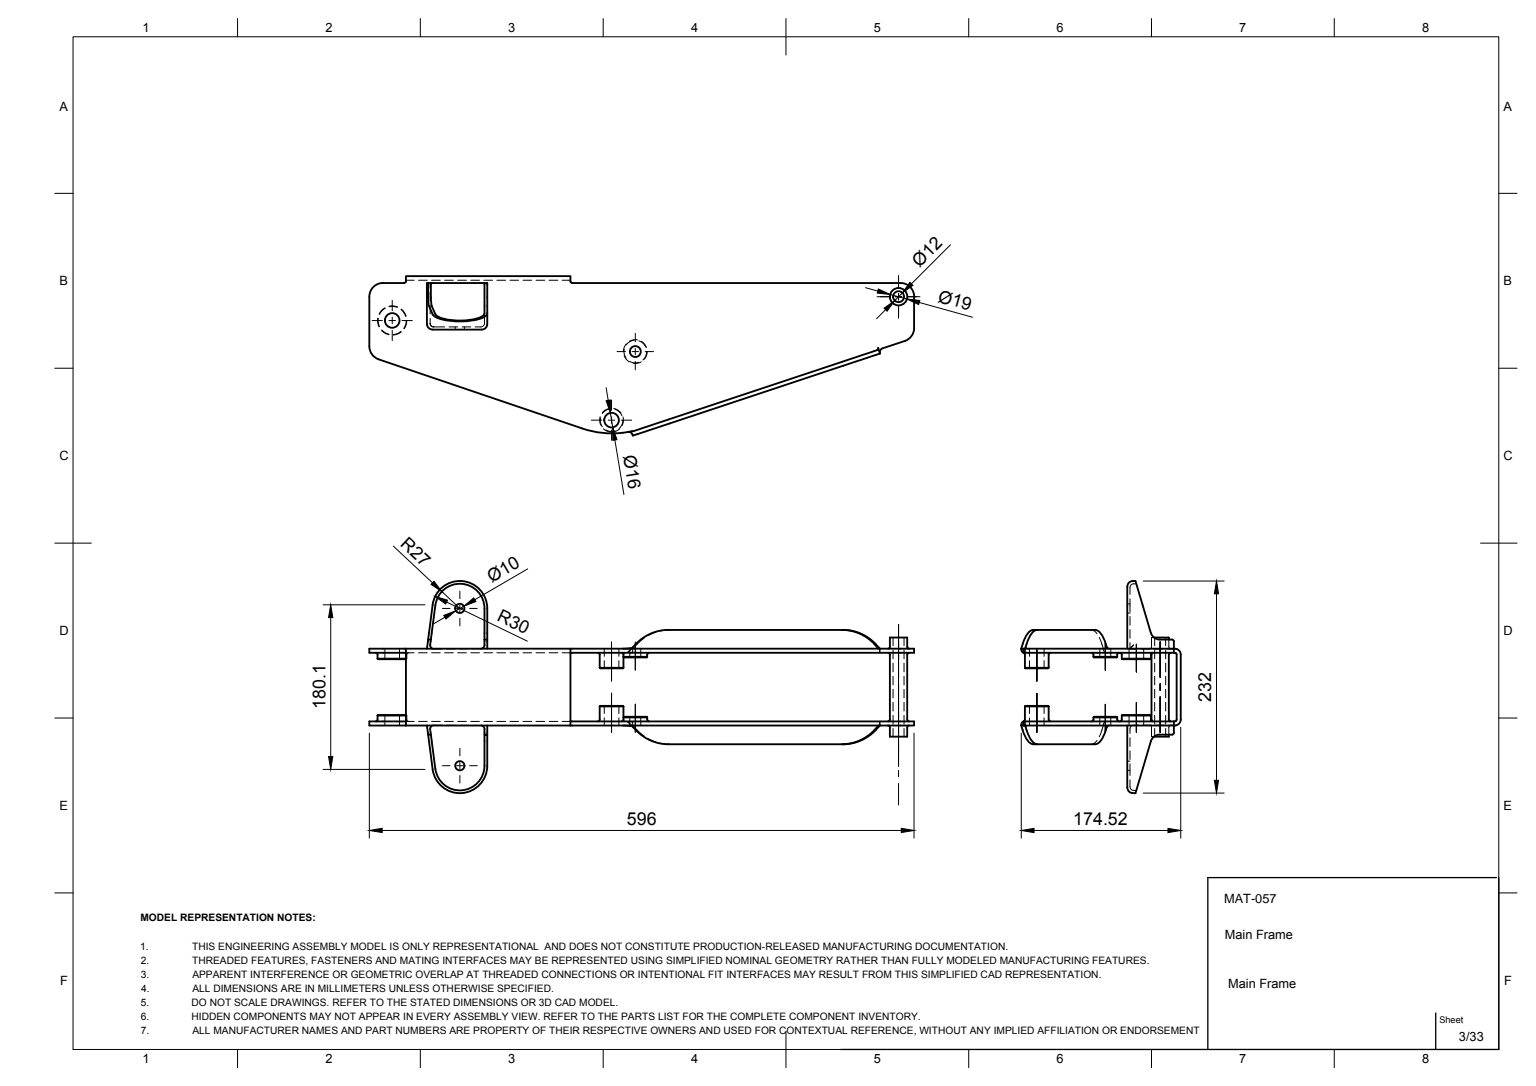
ISO-10303-21;
HEADER;
/* Generated by software containing ST-Developer
 * from STEP Tools, Inc. (www.steptools.com) 
 */

FILE_DESCRIPTION(
/* description */ ('STEP AP214', 'CAx-IF Rec.Pracs.---Representation and Presentation of Product Manufa
cturing Information (PMI)---4.0---2014-10-13'),
/* implementation_level */ '2;1');

FILE_NAME(
/* name */ 'Main Frame.step',
/* time_stamp */ '2026-10-28T23:34:22+01:00',
/* author */ (''),
/* organization */ (''),
/* preprocessor_version */ 'ST-DEVELOPER v20.2',
/* originating_system */ 'Autodesk Translation Framework v15.17.0.0',
/* authorisation */ '');

FILE_SCHEMA (('AP242_MANAGED_MODEL_BASED_3D_ENGINEERING_MIM_LF { 1 0 10303 442 2 1 4 }'));
ENDSEC;

DATA;
#10=MECHANICAL_DESIGN_GEOMETRIC_PRESENTATION_REPRESENTATION('',(#250),#27807);
#206=SHAPE_REPRESENTATION_RELATIONSHIP('SRR','None',#27900,#228);
#228=ADVANCED_BREP_SHAPE_REPRESENTATION('',(#279),#27780);
#250=STYLED_ITEM('',(#28056),#279);
#279=MANIFOLD_SOLID_BREP('Body1',#12026);
#308=(
BOUNDED_SURFACE()
B_SPLINE_SURFACE(3,2,((#18358,#18359,#18360),(#18361,#18362,#18363),(#18364,
#18365,#18366),(#18367,#18368,#18369),(#18370,#18371,#18372),(#18373,#18374,
#18375),(#18376,#18377,#18378),(#18379,#18380,#18381),(#18382,#18383,#18384),
(#18385,#18386,#18387),(#18388,#18389,#18390),(#18391,#18392,#18393)),
 .UNSPECIFIED.,.F.,.F.,.F.)
B_SPLINE_SURFACE_WITH_KNOTS((4,2,2,2,2,4),(3,3),(0.00614272984621533,0.00826669470830694,
0.0093243666888766,0.0103820386694462,0.0124973826305856,0.0146213474926772),
(-5.56138348356354E-6,1.00000862090095),.UNSPECIFIED.)
GEOMETRIC_REPRESENTATION_ITEM()
RATIONAL_B_SPLINE_SURFACE(((1.00000326161464,0.706759768309428,1.00000505596187),
(1.00000294808663,0.734947962870916,1.0000045699493),(1.00000271960407,
0.755490020803058,1.00000421576918),(1.00000249159586,0.775989432119934,
1.00000386232436),(1.00000243486445,0.781089952812372,1.00000377438268),
(1.00000236001445,0.787819451076599,1.00000365835465),(1.00000234158956,
0.789475967918314,1.00000362979347),(1.00000234175209,0.789461355655222,
1.00000363004541),(1.00000241511518,0.782865540172825,1.00000374376852),
(1.00000271619428,0.755796583331183,1.00000421048352),(1.00000294648698,
0.73509178111339,1.00000456746963),(1.00000326163437,0.706757994665561,
1.00000505599245)))
REPRESENTATION_ITEM('')
SURFACE()
);
#309=(
BOUNDED_SURFACE()
B_SPLINE_SURFACE(3,2,((#18394,#18395,#18396),(#18397,#18398,#18399),(#18400,
#18401,#18402),(#18403,#18404,#18405),(#18406,#18407,#18408),(#18409,#18410,
#18411),(#18412,#18413,#18414),(#18415,#18416,#18417),(#18418,#18419,#18420),
(#18421,#18422,#18423),(#18424,#18425,#18426),(#18427,#18428,#18429)),
 .UNSPECIFIED.,.F.,.F.,.F.)
B_SPLINE_SURFACE_WITH_KNOTS((4,2,2,2,2,4),(3,3),(0.0061427298469283,0.00826669470830711,
0.00932436668887678,0.0103820386694465,0.0124973826305858,0.0146213474919646),
(-5.56138389865551E-6,1.00000862090024),.UNSPECIFIED.)
GEOMETRIC_REPRESENTATION_ITEM()
RATIONAL_B_SPLINE_SURFACE(((1.00000326161489,0.706759768337872,1.00000505596145),
(1.00000294808685,0.734947962886857,1.00000456994892),(1.00000271960428,
0.755490020804993,1.00000421576883),(1.00000249159605,0.775989432121355,
1.00000386232404),(1.00000243486463,0.781089952811801,1.00000377438237),
(1.00000236001463,0.787819451077305,1.00000365835434),(1.00000234158974,
0.789475967918561,1.00000362979317),(1.00000234175227,0.789461355654949,
1.00000363004511),(1.00000241511536,0.782865540177451,1.00000374376821),
(1.00000271619448,0.755796583331235,1.00000421048317),(1.0000029464872,
0.735091781130856,1.00000456746925),(1.00000326163462,0.706757994694133,
1.00000505599203)))
REPRESENTATION_ITEM('')
SURFACE()
);
#327=SPHERICAL_SURFACE('',#12617,4.);
#328=SPHERICAL_SURFACE('',#12619,4.);
#335=FACE_BOUND('',#2001,.T.);
#336=FACE_BOUND('',#2002,.T.);
#337=FACE_BOUND('',#2003,.T.);
#338=FACE_BOUND('',#2004,.T.);
#339=FACE_BOUND('',#2005,.T.);
#340=FACE_BOUND('',#2007,.T.);
#341=FACE_BOUND('',#2008,.T.);
#342=FACE_BOUND('',#2009,.T.);
#343=FACE_BOUND('',#2014,.T.);
#344=FACE_BOUND('',#2015,.T.);
#345=FACE_BOUND('',#2016,.T.);
#346=FACE_BOUND('',#2017,.T.);
#347=FACE_BOUND('',#2018,.T.);
#348=FACE_BOUND('',#2024,.T.);
#349=FACE_BOUND('',#2029,.T.);
#350=FACE_BOUND('',#2034,.T.);
#351=FACE_BOUND('',#2051,.T.);
#352=FACE_BOUND('',#2053,.T.);
#353=FACE_BOUND('',#2055,.T.);
#354=FACE_BOUND('',#2061,.T.);
#355=FACE_BOUND('',#2062,.T.);
#356=FACE_BOUND('',#2063,.T.);
#357=FACE_BOUND('',#2065,.T.);
#358=FACE_BOUND('',#2067,.T.);
#359=FACE_BOUND('',#2072,.T.);
#360=FACE_BOUND('',#2083,.T.);
#361=FACE_BOUND('',#2085,.T.);
#362=FACE_BOUND('',#2087,.T.);
#448=PLANE('',#12425);
#449=PLANE('',#12427);
#450=PLANE('',#12428);
#451=PLANE('',#12429);
#452=PLANE('',#12431);
#453=PLANE('',#12432);
#454=PLANE('',#12440);
#455=PLANE('',#12443);
#456=PLANE('',#12444);
#457=PLANE('',#12451);
#458=PLANE('',#12452);
#459=PLANE('',#12453);
#460=PLANE('',#12455);
#461=PLANE('',#12457);
#462=PLANE('',#12466);
#463=PLANE('',#12477);
#464=PLANE('',#12478);
#465=PLANE('',#12482);
#466=PLANE('',#12493);
#467=PLANE('',#12494);
#468=PLANE('',#12495);
#469=PLANE('',#12496);
#470=PLANE('',#12497);
#471=PLANE('',#12498);
#472=PLANE('',#12503);
#473=PLANE('',#12506);
#474=PLANE('',#12508);
#475=PLANE('',#12511);
#476=PLANE('',#12513);
#477=PLANE('',#12515);
#478=PLANE('',#12519);
#479=PLANE('',#12521);
#480=PLANE('',#12529);
#481=PLANE('',#12530);
#482=PLANE('',#12533);
#483=PLANE('',#12535);
#484=PLANE('',#12537);
#485=PLANE('',#12540);
#486=PLANE('',#12543);
#487=PLANE('',#12544);
#488=PLANE('',#12545);
#489=PLANE('',#12546);
#490=PLANE('',#12547);
#491=PLANE('',#12548);
#492=PLANE('',#12549);
#493=PLANE('',#12550);
#494=PLANE('',#12558);
#495=PLANE('',#12559);
#496=PLANE('',#12560);
#497=PLANE('',#12562);
#498=PLANE('',#12564);
#499=PLANE('',#12566);
#500=PLANE('',#12571);
#501=PLANE('',#12573);
#502=PLANE('',#12576);
#503=PLANE('',#12577);
#504=PLANE('',#12579);
#505=PLANE('',#12582);
#506=PLANE('',#12583);
#507=PLANE('',#12584);
#508=PLANE('',#12585);
#509=PLANE('',#12588);
#510=PLANE('',#12589);
#511=PLANE('',#12591);
#512=PLANE('',#12592);
#513=PLANE('',#12597);
#747=ELLIPSE('',#12376,5.6568542494854,3.99999999999488);
#748=ELLIPSE('',#12390,28.164698545175,26.9999999999996);
#749=ELLIPSE('',#12421,31.2941094946442,30.0000000000042);
#750=ELLIPSE('',#12435,141.421352252718,99.9999944851797);
#751=ELLIPSE('',#12449,10.0848897519878,9.99999999999638);
#752=ELLIPSE('',#12450,10.0848897519895,9.99999999999823);
#753=ELLIPSE('',#12456,2.01697795039841,2.0000000000002);
#754=ELLIPSE('',#12465,6.05093385119014,5.9999999999955);
#755=ELLIPSE('',#12492,6.05093385118888,5.99999999999402);
#756=ELLIPSE('',#12502,31.2941094946394,29.9999999999999);
#757=ELLIPSE('',#12504,10.0848897519875,9.99999999999656);
#758=ELLIPSE('',#12505,2.01697795039468,1.99999999999602);
#759=ELLIPSE('',#12510,10.084889751988,9.99999999999652);
#760=ELLIPSE('',#12512,28.1646985451758,27.);
#761=ELLIPSE('',#12520,2.01697795039476,1.99999999999607);
#762=ELLIPSE('',#12523,141.421350791142,99.9999924642367);
#763=ELLIPSE('',#12534,2.82842712474556,1.9999999999995);
#764=ELLIPSE('',#12538,2.8284271247638,2.00000000001808);
#765=ELLIPSE('',#12539,6.36396103068019,4.50000000000073);
#766=ELLIPSE('',#12561,4.00607672981957,4.00312101599644);
#767=ELLIPSE('',#12565,2.01697795039961,2.00000000000168);
#768=ELLIPSE('',#12574,6.36396103067894,4.49999999999996);
#769=ELLIPSE('',#12575,2.82842712478915,2.00000000005605);
#770=ELLIPSE('',#12578,2.82842712474301,1.99999999999741);
#771=ELLIPSE('',#12607,5.65685424949513,4.00000000000238);
#811=TOROIDAL_SURFACE('',#12321,24.,6.);
#812=TOROIDAL_SURFACE('',#12326,18.,2.);
#813=TOROIDAL_SURFACE('',#12330,15.,2.);
#814=TOROIDAL_SURFACE('',#12334,15.,2.);
#815=TOROIDAL_SURFACE('',#12338,18.,2.);
#816=TOROIDAL_SURFACE('',#12342,15.,2.);
#817=TOROIDAL_SURFACE('',#12348,15.,2.);
#818=TOROIDAL_SURFACE('',#12354,11.5,2.);
#819=TOROIDAL_SURFACE('',#12359,11.5,2.);
#820=TOROIDAL_SURFACE('',#12363,11.5,2.);
#821=TOROIDAL_SURFACE('',#12368,11.5,2.);
#822=TOROIDAL_SURFACE('',#12378,23.,4.);
#823=TOROIDAL_SURFACE('',#12625,23.,4.);
#824=TOROIDAL_SURFACE('',#12640,24.,6.);
#850=B_SPLINE_CURVE_WITH_KNOTS('',3,(#17467,#17468,#17469,#17470,#17471,
#17472,#17473,#17474,#17475,#17476,#17477,#17478),.UNSPECIFIED.,.F.,.F.,
(4,2,2,2,2,4),(2.0099992972745,2.20224824152656,2.28793503314165,2.37362182475674,
2.53832634192652,2.7030308590963),.UNSPECIFIED.);
#851=B_SPLINE_CURVE_WITH_KNOTS('',3,(#17597,#17598,#17599,#17600,#17601,
#17602,#17603,#17604,#17605,#17606,#17607,#17608),.UNSPECIFIED.,.F.,.F.,
(4,2,2,2,2,4),(0.,0.00181440406025865,0.00272160609038796,0.00362880812051727,
0.00544321218077591,0.00725761624103455),.UNSPECIFIED.);
#852=B_SPLINE_CURVE_WITH_KNOTS('',3,(#17643,#17644,#17645,#17646,#17647,
#17648,#17649,#17650,#17651,#17652,#17653,#17654),.UNSPECIFIED.,.F.,.F.,
(4,2,2,2,2,4),(0.,0.00181440406025865,0.00272160609038798,0.0036288081205173,
0.00544321218077593,0.00725761624103456),.UNSPECIFIED.);
#853=B_SPLINE_CURVE_WITH_KNOTS('',3,(#17772,#17773,#17774,#17775,#17776,
#17777),.UNSPECIFIED.,.F.,.F.,(4,2,4),(-1.89448158063908,-0.947240790319523,
-0.943407967638861),.UNSPECIFIED.);
#854=B_SPLINE_CURVE_WITH_KNOTS('',3,(#18063,#18064,#18065,#18066,#18067,
#18068),.UNSPECIFIED.,.F.,.F.,(4,2,4),(-4.54637383394205,-4.54254101126139,
-3.59530022094183),.UNSPECIFIED.);
#855=B_SPLINE_CURVE_WITH_KNOTS('',3,(#18285,#18286,#18287,#18288,#18289,
#18290,#18291,#18292,#18293,#18294),.UNSPECIFIED.,.F.,.F.,(4,2,2,2,4),(-1.65528023567133,
-1.60355895330957,-1.50636781568743,-1.40917667806529,-1.31726787147769),
 .UNSPECIFIED.);
#856=B_SPLINE_CURVE_WITH_KNOTS('',3,(#18296,#18297,#18298,#18299,#18300,
#18301,#18302,#18303,#18304,#18305),.UNSPECIFIED.,.F.,.F.,(4,2,2,2,4),(-0.723638776454986,
-0.631729969867392,-0.53453883224525,-0.437347694623109,-0.385626412261347),
 .UNSPECIFIED.);
#857=B_SPLINE_CURVE_WITH_KNOTS('',3,(#18306,#18307,#18308,#18309,#18310,
#18311,#18312,#18313,#18314,#18315,#18316,#18317),.UNSPECIFIED.,.F.,.F.,
(4,2,2,2,2,4),(0.207978724543637,0.400227668795699,0.48591446041079,0.57160125202588,
0.736305769195657,0.901010286365433),.UNSPECIFIED.);
#858=B_SPLINE_CURVE_WITH_KNOTS('',3,(#18319,#18320,#18321,#18322,#18323,
#18324,#18325,#18326),.UNSPECIFIED.,.F.,.F.,(4,2,2,4),(0.724350563126704,
0.774624716441459,0.824898869756215,0.828883959825179),.UNSPECIFIED.);
#859=B_SPLINE_CURVE_WITH_KNOTS('',3,(#18327,#18328,#18329,#18330,#18331,
#18332,#18333,#18334),.UNSPECIFIED.,.F.,.F.,(4,2,2,4),(1.23194128218264,
1.2359263722516,1.28620052556636,1.33647467888111),.UNSPECIFIED.);
#860=B_SPLINE_CURVE_WITH_KNOTS('',3,(#18336,#18337,#18338,#18339,#18340,
#18341,#18342,#18343),.UNSPECIFIED.,.F.,.F.,(4,2,2,4),(-0.306062057877202,
-0.255787904562446,-0.205513751247691,-0.201528661178732),.UNSPECIFIED.);
#861=B_SPLINE_CURVE_WITH_KNOTS('',3,(#18344,#18345,#18346,#18347,#18348,
#18349,#18350,#18351),.UNSPECIFIED.,.F.,.F.,(4,2,2,4),(0.201528661178729,
0.205513751247691,0.255787904562446,0.306062057877201),.UNSPECIFIED.);
#862=B_SPLINE_CURVE_WITH_KNOTS('',3,(#18438,#18439,#18440,#18441,#18442,
#18443),.UNSPECIFIED.,.F.,.F.,(4,2,4),(-0.302135903177322,-0.22673410522417,
-0.201580663771353),.UNSPECIFIED.);
#863=B_SPLINE_CURVE_WITH_KNOTS('',3,(#18445,#18446,#18447,#18448,#18449,
#18450),.UNSPECIFIED.,.F.,.F.,(4,2,4),(-0.409607477693974,-0.384454036241157,
-0.309052238288002),.UNSPECIFIED.);
#864=B_SPLINE_CURVE_WITH_KNOTS('',3,(#18452,#18453,#18454,#18455,#18456,
#18457),.UNSPECIFIED.,.F.,.F.,(4,2,4),(-0.302135903177326,-0.226734105224171,
-0.201580663771353),.UNSPECIFIED.);
#865=B_SPLINE_CURVE_WITH_KNOTS('',3,(#18459,#18460,#18461,#18462,#18463,
#18464),.UNSPECIFIED.,.F.,.F.,(4,2,4),(-0.409607477693974,-0.384454036241154,
-0.309052238288002),.UNSPECIFIED.);
#975=CYLINDRICAL_SURFACE('',#12318,4.5);
#976=CYLINDRICAL_SURFACE('',#12373,4.);
#977=CYLINDRICAL_SURFACE('',#12383,6.00000000000001);
#978=CYLINDRICAL_SURFACE('',#12386,13.);
#979=CYLINDRICAL_SURFACE('',#12387,13.);
#980=CYLINDRICAL_SURFACE('',#12388,16.);
#981=CYLINDRICAL_SURFACE('',#12389,27.);
#982=CYLINDRICAL_SURFACE('',#12391,9.50000000000001);
#983=CYLINDRICAL_SURFACE('',#12393,5.99999999999999);
#984=CYLINDRICAL_SURFACE('',#12396,8.00000000000001);
#985=CYLINDRICAL_SURFACE('',#12399,7.99999999999999);
#986=CYLINDRICAL_SURFACE('',#12402,13.);
#987=CYLINDRICAL_SURFACE('',#12403,13.);
#988=CYLINDRICAL_SURFACE('',#12404,16.);
#989=CYLINDRICAL_SURFACE('',#12405,9.50000000000001);
#990=CYLINDRICAL_SURFACE('',#12407,5.99999999999999);
#991=CYLINDRICAL_SURFACE('',#12410,8.00000000000001);
#992=CYLINDRICAL_SURFACE('',#12413,7.99999999999999);
#993=CYLINDRICAL_SURFACE('',#12416,9.50000000000001);
#994=CYLINDRICAL_SURFACE('',#12417,5.);
#995=CYLINDRICAL_SURFACE('',#12420,30.);
#996=CYLINDRICAL_SURFACE('',#12422,5.);
#997=CYLINDRICAL_SURFACE('',#12434,100.);
#998=CYLINDRICAL_SURFACE('',#12445,10.);
#999=CYLINDRICAL_SURFACE('',#12448,10.);
#1000=CYLINDRICAL_SURFACE('',#12479,10.);
#1001=CYLINDRICAL_SURFACE('',#12500,30.);
#1002=CYLINDRICAL_SURFACE('',#12509,10.);
#1003=CYLINDRICAL_SURFACE('',#12517,27.);
#1004=CYLINDRICAL_SURFACE('',#12522,100.);
#1005=CYLINDRICAL_SURFACE('',#12525,15.);
#1006=CYLINDRICAL_SURFACE('',#12526,15.);
#1007=CYLINDRICAL_SURFACE('',#12527,15.);
#1008=CYLINDRICAL_SURFACE('',#12528,15.);
#1009=CYLINDRICAL_SURFACE('',#12567,15.);
#1010=CYLINDRICAL_SURFACE('',#12568,15.);
#1011=CYLINDRICAL_SURFACE('',#12569,15.);
#1012=CYLINDRICAL_SURFACE('',#12570,15.);
#1013=CYLINDRICAL_SURFACE('',#12602,53.);
#1014=CYLINDRICAL_SURFACE('',#12603,53.);
#1015=CYLINDRICAL_SURFACE('',#12604,53.);
#1016=CYLINDRICAL_SURFACE('',#12605,53.);
#1017=CYLINDRICAL_SURFACE('',#12606,4.);
#1018=CYLINDRICAL_SURFACE('',#12608,4.);
#1019=CYLINDRICAL_SURFACE('',#12609,4.00000000000001);
#1020=CYLINDRICAL_SURFACE('',#12610,4.);
#1021=CYLINDRICAL_SURFACE('',#12612,4.);
#1022=CYLINDRICAL_SURFACE('',#12614,3.99999999999998);
#1023=CYLINDRICAL_SURFACE('',#12621,4.);
#1024=CYLINDRICAL_SURFACE('',#12623,4.);
#1025=CYLINDRICAL_SURFACE('',#12626,4.);
#1026=CYLINDRICAL_SURFACE('',#12627,4.);
#1027=CYLINDRICAL_SURFACE('',#12628,2.);
#1028=CYLINDRICAL_SURFACE('',#12629,2.);
#1029=CYLINDRICAL_SURFACE('',#12630,2.);
#1030=CYLINDRICAL_SURFACE('',#12631,2.);
#1031=CYLINDRICAL_SURFACE('',#12632,1.99999999999999);
#1032=CYLINDRICAL_SURFACE('',#12633,1.99999999999999);
#1033=CYLINDRICAL_SURFACE('',#12634,2.);
#1034=CYLINDRICAL_SURFACE('',#12635,2.);
#1035=CYLINDRICAL_SURFACE('',#12636,6.00000000000001);
#1036=CYLINDRICAL_SURFACE('',#12637,5.99999999999999);
#1037=CYLINDRICAL_SURFACE('',#12638,6.00000000000001);
#1038=CYLINDRICAL_SURFACE('',#12642,5.99999999999999);
#1039=CYLINDRICAL_SURFACE('',#12643,2.);
#1040=CYLINDRICAL_SURFACE('',#12644,2.);
#1041=CYLINDRICAL_SURFACE('',#12645,2.);
#1042=CYLINDRICAL_SURFACE('',#12646,2.);
#1043=CYLINDRICAL_SURFACE('',#12647,4.5);
#1044=CYLINDRICAL_SURFACE('',#12648,4.5);
#1045=CYLINDRICAL_SURFACE('',#12649,4.5);
#1046=CYLINDRICAL_SURFACE('',#12650,6.50000000000001);
#1047=CYLINDRICAL_SURFACE('',#12651,6.50000000000001);
#1247=FACE_OUTER_BOUND('',#1944,.T.);
#1248=FACE_OUTER_BOUND('',#1945,.T.);
#1249=FACE_OUTER_BOUND('',#1946,.T.);
#1250=FACE_OUTER_BOUND('',#1947,.T.);
#1251=FACE_OUTER_BOUND('',#1948,.T.);
#1252=FACE_OUTER_BOUND('',#1949,.T.);
#1253=FACE_OUTER_BOUND('',#1950,.T.);
#1254=FACE_OUTER_BOUND('',#1951,.T.);
#1255=FACE_OUTER_BOUND('',#1952,.T.);
#1256=FACE_OUTER_BOUND('',#1953,.T.);
#1257=FACE_OUTER_BOUND('',#1954,.T.);
#1258=FACE_OUTER_BOUND('',#1955,.T.);
#1259=FACE_OUTER_BOUND('',#1956,.T.);
#1260=FACE_OUTER_BOUND('',#1957,.T.);
#1261=FACE_OUTER_BOUND('',#1958,.T.);
#1262=FACE_OUTER_BOUND('',#1959,.T.);
#1263=FACE_OUTER_BOUND('',#1960,.T.);
#1264=FACE_OUTER_BOUND('',#1961,.T.);
#1265=FACE_OUTER_BOUND('',#1962,.T.);
#1266=FACE_OUTER_BOUND('',#1963,.T.);
#1267=FACE_OUTER_BOUND('',#1964,.T.);
#1268=FACE_OUTER_BOUND('',#1965,.T.);
#1269=FACE_OUTER_BOUND('',#1966,.T.);
#1270=FACE_OUTER_BOUND('',#1967,.T.);
#1271=FACE_OUTER_BOUND('',#1968,.T.);
#1272=FACE_OUTER_BOUND('',#1969,.T.);
#1273=FACE_OUTER_BOUND('',#1970,.T.);
#1274=FACE_OUTER_BOUND('',#1971,.T.);
#1275=FACE_OUTER_BOUND('',#1972,.T.);
#1276=FACE_OUTER_BOUND('',#1973,.T.);
#1277=FACE_OUTER_BOUND('',#1974,.T.);
#1278=FACE_OUTER_BOUND('',#1975,.T.);
#1279=FACE_OUTER_BOUND('',#1976,.T.);
#1280=FACE_OUTER_BOUND('',#1977,.T.);
#1281=FACE_OUTER_BOUND('',#1978,.T.);
#1282=FACE_OUTER_BOUND('',#1979,.T.);
#1283=FACE_OUTER_BOUND('',#1980,.T.);
#1284=FACE_OUTER_BOUND('',#1981,.T.);
#1285=FACE_OUTER_BOUND('',#1982,.T.);
#1286=FACE_OUTER_BOUND('',#1983,.T.);
#1287=FACE_OUTER_BOUND('',#1984,.T.);
#1288=FACE_OUTER_BOUND('',#1985,.T.);
#1289=FACE_OUTER_BOUND('',#1986,.T.);
#1290=FACE_OUTER_BOUND('',#1987,.T.);
#1291=FACE_OUTER_BOUND('',#1988,.T.);
#1292=FACE_OUTER_BOUND('',#1989,.T.);
#1293=FACE_OUTER_BOUND('',#1990,.T.);
#1294=FACE_OUTER_BOUND('',#1991,.T.);
#1295=FACE_OUTER_BOUND('',#1992,.T.);
#1296=FACE_OUTER_BOUND('',#1993,.T.);
#1297=FACE_OUTER_BOUND('',#1994,.T.);
#1298=FACE_OUTER_BOUND('',#1995,.T.);
#1299=FACE_OUTER_BOUND('',#1996,.T.);
#1300=FACE_OUTER_BOUND('',#1997,.T.);
#1301=FACE_OUTER_BOUND('',#1998,.T.);
#1302=FACE_OUTER_BOUND('',#1999,.T.);
#1303=FACE_OUTER_BOUND('',#2000,.T.);
#1304=FACE_OUTER_BOUND('',#2006,.T.);
#1305=FACE_OUTER_BOUND('',#2010,.T.);
#1306=FACE_OUTER_BOUND('',#2011,.T.);
#1307=FACE_OUTER_BOUND('',#2012,.T.);
#1308=FACE_OUTER_BOUND('',#2013,.T.);
#1309=FACE_OUTER_BOUND('',#2019,.T.);
#1310=FACE_OUTER_BOUND('',#2020,.T.);
#1311=FACE_OUTER_BOUND('',#2021,.T.);
#1312=FACE_OUTER_BOUND('',#2022,.T.);
#1313=FACE_OUTER_BOUND('',#2023,.T.);
#1314=FACE_OUTER_BOUND('',#2025,.T.);
#1315=FACE_OUTER_BOUND('',#2026,.T.);
#1316=FACE_OUTER_BOUND('',#2027,.T.);
#1317=FACE_OUTER_BOUND('',#2028,.T.);
#1318=FACE_OUTER_BOUND('',#2030,.T.);
#1319=FACE_OUTER_BOUND('',#2031,.T.);
#1320=FACE_OUTER_BOUND('',#2032,.T.);
#1321=FACE_OUTER_BOUND('',#2033,.T.);
#1322=FACE_OUTER_BOUND('',#2035,.T.);
#1323=FACE_OUTER_BOUND('',#2036,.T.);
#1324=FACE_OUTER_BOUND('',#2037,.T.);
#1325=FACE_OUTER_BOUND('',#2038,.T.);
#1326=FACE_OUTER_BOUND('',#2039,.T.);
#1327=FACE_OUTER_BOUND('',#2040,.T.);
#1328=FACE_OUTER_BOUND('',#2041,.T.);
#1329=FACE_OUTER_BOUND('',#2042,.T.);
#1330=FACE_OUTER_BOUND('',#2043,.T.);
#1331=FACE_OUTER_BOUND('',#2044,.T.);
#1332=FACE_OUTER_BOUND('',#2045,.T.);
#1333=FACE_OUTER_BOUND('',#2046,.T.);
#1334=FACE_OUTER_BOUND('',#2047,.T.);
#1335=FACE_OUTER_BOUND('',#2048,.T.);
#1336=FACE_OUTER_BOUND('',#2049,.T.);
#1337=FACE_OUTER_BOUND('',#2050,.T.);
#1338=FACE_OUTER_BOUND('',#2052,.T.);
#1339=FACE_OUTER_BOUND('',#2054,.T.);
#1340=FACE_OUTER_BOUND('',#2056,.T.);
#1341=FACE_OUTER_BOUND('',#2057,.T.);
#1342=FACE_OUTER_BOUND('',#2058,.T.);
#1343=FACE_OUTER_BOUND('',#2059,.T.);
#1344=FACE_OUTER_BOUND('',#2060,.T.);
#1345=FACE_OUTER_BOUND('',#2064,.T.);
#1346=FACE_OUTER_BOUND('',#2066,.T.);
#1347=FACE_OUTER_BOUND('',#2068,.T.);
#1348=FACE_OUTER_BOUND('',#2069,.T.);
#1349=FACE_OUTER_BOUND('',#2070,.T.);
#1350=FACE_OUTER_BOUND('',#2071,.T.);
#1351=FACE_OUTER_BOUND('',#2073,.T.);
#1352=FACE_OUTER_BOUND('',#2074,.T.);
#1353=FACE_OUTER_BOUND('',#2075,.T.);
#1354=FACE_OUTER_BOUND('',#2076,.T.);
#1355=FACE_OUTER_BOUND('',#2077,.T.);
#1356=FACE_OUTER_BOUND('',#2078,.T.);
#1357=FACE_OUTER_BOUND('',#2079,.T.);
#1358=FACE_OUTER_BOUND('',#2080,.T.);
#1359=FACE_OUTER_BOUND('',#2081,.T.);
#1360=FACE_OUTER_BOUND('',#2082,.T.);
#1361=FACE_OUTER_BOUND('',#2084,.T.);
#1362=FACE_OUTER_BOUND('',#2086,.T.);
#1363=FACE_OUTER_BOUND('',#2088,.T.);
#1364=FACE_OUTER_BOUND('',#2089,.T.);
#1365=FACE_OUTER_BOUND('',#2090,.T.);
#1366=FACE_OUTER_BOUND('',#2091,.T.);
#1367=FACE_OUTER_BOUND('',#2092,.T.);
#1368=FACE_OUTER_BOUND('',#2093,.T.);
#1369=FACE_OUTER_BOUND('',#2094,.T.);
#1370=FACE_OUTER_BOUND('',#2095,.T.);
#1371=FACE_OUTER_BOUND('',#2096,.T.);
#1372=FACE_OUTER_BOUND('',#2097,.T.);
#1373=FACE_OUTER_BOUND('',#2098,.T.);
#1374=FACE_OUTER_BOUND('',#2099,.T.);
#1375=FACE_OUTER_BOUND('',#2100,.T.);
#1376=FACE_OUTER_BOUND('',#2101,.T.);
#1377=FACE_OUTER_BOUND('',#2102,.T.);
#1378=FACE_OUTER_BOUND('',#2103,.T.);
#1379=FACE_OUTER_BOUND('',#2104,.T.);
#1380=FACE_OUTER_BOUND('',#2105,.T.);
#1381=FACE_OUTER_BOUND('',#2106,.T.);
#1382=FACE_OUTER_BOUND('',#2107,.T.);
#1383=FACE_OUTER_BOUND('',#2108,.T.);
#1384=FACE_OUTER_BOUND('',#2109,.T.);
#1385=FACE_OUTER_BOUND('',#2110,.T.);
#1386=FACE_OUTER_BOUND('',#2111,.T.);
#1387=FACE_OUTER_BOUND('',#2112,.T.);
#1388=FACE_OUTER_BOUND('',#2113,.T.);
#1389=FACE_OUTER_BOUND('',#2114,.T.);
#1390=FACE_OUTER_BOUND('',#2115,.T.);
#1391=FACE_OUTER_BOUND('',#2116,.T.);
#1392=FACE_OUTER_BOUND('',#2117,.T.);
#1393=FACE_OUTER_BOUND('',#2118,.T.);
#1394=FACE_OUTER_BOUND('',#2119,.T.);
#1395=FACE_OUTER_BOUND('',#2120,.T.);
#1396=FACE_OUTER_BOUND('',#2121,.T.);
#1397=FACE_OUTER_BOUND('',#2122,.T.);
#1398=FACE_OUTER_BOUND('',#2123,.T.);
#1399=FACE_OUTER_BOUND('',#2124,.T.);
#1400=FACE_OUTER_BOUND('',#2125,.T.);
#1401=FACE_OUTER_BOUND('',#2126,.T.);
#1402=FACE_OUTER_BOUND('',#2127,.T.);
#1403=FACE_OUTER_BOUND('',#2128,.T.);
#1404=FACE_OUTER_BOUND('',#2129,.T.);
#1405=FACE_OUTER_BOUND('',#2130,.T.);
#1406=FACE_OUTER_BOUND('',#2131,.T.);
#1407=FACE_OUTER_BOUND('',#2132,.T.);
#1408=FACE_OUTER_BOUND('',#2133,.T.);
#1409=FACE_OUTER_BOUND('',#2134,.T.);
#1944=EDGE_LOOP('',(#7851,#7852,#7853,#7854));
#1945=EDGE_LOOP('',(#7855,#7856,#7857,#7858));
#1946=EDGE_LOOP('',(#7859,#7860,#7861,#7862));
#1947=EDGE_LOOP('',(#7863,#7864,#7865,#7866));
#1948=EDGE_LOOP('',(#7867,#7868,#7869,#7870));
#1949=EDGE_LOOP('',(#7871,#7872,#7873,#7874));
#1950=EDGE_LOOP('',(#7875,#7876,#7877,#7878,#7879));
#1951=EDGE_LOOP('',(#7880,#7881,#7882,#7883));
#1952=EDGE_LOOP('',(#7884,#7885,#7886,#7887));
#1953=EDGE_LOOP('',(#7888,#7889,#7890,#7891));
#1954=EDGE_LOOP('',(#7892,#7893,#7894,#7895));
#1955=EDGE_LOOP('',(#7896,#7897,#7898,#7899));
#1956=EDGE_LOOP('',(#7900,#7901,#7902,#7903,#7904));
#1957=EDGE_LOOP('',(#7905,#7906,#7907,#7908,#7909));
#1958=EDGE_LOOP('',(#7910,#7911,#7912,#7913,#7914));
#1959=EDGE_LOOP('',(#7915,#7916,#7917,#7918));
#1960=EDGE_LOOP('',(#7919,#7920,#7921,#7922,#7923));
#1961=EDGE_LOOP('',(#7924,#7925,#7926,#7927,#7928));
#1962=EDGE_LOOP('',(#7929,#7930,#7931,#7932,#7933,#7934));
#1963=EDGE_LOOP('',(#7935,#7936,#7937,#7938));
#1964=EDGE_LOOP('',(#7939,#7940,#7941,#7942));
#1965=EDGE_LOOP('',(#7943,#7944,#7945,#7946));
#1966=EDGE_LOOP('',(#7947,#7948,#7949,#7950,#7951,#7952));
#1967=EDGE_LOOP('',(#7953,#7954,#7955,#7956));
#1968=EDGE_LOOP('',(#7957,#7958,#7959,#7960));
#1969=EDGE_LOOP('',(#7961,#7962,#7963,#7964,#7965));
#1970=EDGE_LOOP('',(#7966,#7967,#7968,#7969));
#1971=EDGE_LOOP('',(#7970,#7971,#7972,#7973));
#1972=EDGE_LOOP('',(#7974,#7975,#7976,#7977));
#1973=EDGE_LOOP('',(#7978,#7979,#7980,#7981));
#1974=EDGE_LOOP('',(#7982,#7983,#7984,#7985,#7986,#7987));
#1975=EDGE_LOOP('',(#7988,#7989,#7990,#7991));
#1976=EDGE_LOOP('',(#7992,#7993,#7994,#7995,#7996));
#1977=EDGE_LOOP('',(#7997,#7998,#7999,#8000));
#1978=EDGE_LOOP('',(#8001,#8002,#8003,#8004));
#1979=EDGE_LOOP('',(#8005,#8006,#8007,#8008));
#1980=EDGE_LOOP('',(#8009,#8010,#8011,#8012,#8013));
#1981=EDGE_LOOP('',(#8014,#8015,#8016,#8017));
#1982=EDGE_LOOP('',(#8018,#8019,#8020,#8021));
#1983=EDGE_LOOP('',(#8022,#8023,#8024,#8025));
#1984=EDGE_LOOP('',(#8026,#8027,#8028,#8029,#8030));
#1985=EDGE_LOOP('',(#8031,#8032,#8033,#8034));
#1986=EDGE_LOOP('',(#8035,#8036,#8037,#8038,#8039));
#1987=EDGE_LOOP('',(#8040,#8041,#8042,#8043,#8044));
#1988=EDGE_LOOP('',(#8045,#8046,#8047,#8048));
#1989=EDGE_LOOP('',(#8049,#8050,#8051,#8052,#8053));
#1990=EDGE_LOOP('',(#8054,#8055,#8056,#8057,#8058,#8059,#8060,#8061));
#1991=EDGE_LOOP('',(#8062,#8063,#8064,#8065,#8066,#8067));
#1992=EDGE_LOOP('',(#8068,#8069,#8070,#8071));
#1993=EDGE_LOOP('',(#8072,#8073,#8074,#8075,#8076,#8077,#8078,#8079));
#1994=EDGE_LOOP('',(#8080,#8081,#8082,#8083));
#1995=EDGE_LOOP('',(#8084,#8085,#8086,#8087));
#1996=EDGE_LOOP('',(#8088,#8089,#8090,#8091));
#1997=EDGE_LOOP('',(#8092,#8093,#8094,#8095));
#1998=EDGE_LOOP('',(#8096,#8097,#8098,#8099,#8100,#8101,#8102,#8103));
#1999=EDGE_LOOP('',(#8104,#8105,#8106,#8107,#8108,#8109,#8110,#8111));
#2000=EDGE_LOOP('',(#8112,#8113,#8114,#8115,#8116,#8117,#8118,#8119,#8120,
#8121,#8122,#8123,#8124,#8125,#8126,#8127,#8128));
#2001=EDGE_LOOP('',(#8129));
#2002=EDGE_LOOP('',(#8130));
#2003=EDGE_LOOP('',(#8131));
#2004=EDGE_LOOP('',(#8132));
#2005=EDGE_LOOP('',(#8133,#8134,#8135,#8136,#8137,#8138,#8139,#8140));
#2006=EDGE_LOOP('',(#8141,#8142,#8143,#8144,#8145,#8146,#8147,#8148,#8149,
#8150,#8151,#8152,#8153,#8154,#8155,#8156,#8157,#8158,#8159));
#2007=EDGE_LOOP('',(#8160));
#2008=EDGE_LOOP('',(#8161));
#2009=EDGE_LOOP('',(#8162));
#2010=EDGE_LOOP('',(#8163,#8164,#8165,#8166));
#2011=EDGE_LOOP('',(#8167,#8168,#8169,#8170));
#2012=EDGE_LOOP('',(#8171,#8172,#8173,#8174));
#2013=EDGE_LOOP('',(#8175,#8176,#8177,#8178,#8179,#8180,#8181,#8182,#8183,
#8184,#8185,#8186,#8187,#8188,#8189,#8190,#8191));
#2014=EDGE_LOOP('',(#8192));
#2015=EDGE_LOOP('',(#8193));
#2016=EDGE_LOOP('',(#8194));
#2017=EDGE_LOOP('',(#8195));
#2018=EDGE_LOOP('',(#8196,#8197,#8198,#8199,#8200,#8201,#8202,#8203));
#2019=EDGE_LOOP('',(#8204,#8205,#8206,#8207));
#2020=EDGE_LOOP('',(#8208,#8209,#8210,#8211));
#2021=EDGE_LOOP('',(#8212,#8213,#8214,#8215));
#2022=EDGE_LOOP('',(#8216,#8217,#8218,#8219));
#2023=EDGE_LOOP('',(#8220));
#2024=EDGE_LOOP('',(#8221));
#2025=EDGE_LOOP('',(#8222,#8223,#8224,#8225,#8226,#8227,#8228,#8229));
#2026=EDGE_LOOP('',(#8230,#8231,#8232,#8233));
#2027=EDGE_LOOP('',(#8234,#8235,#8236,#8237,#8238,#8239,#8240,#8241));
#2028=EDGE_LOOP('',(#8242,#8243,#8244,#8245));
#2029=EDGE_LOOP('',(#8246));
#2030=EDGE_LOOP('',(#8247,#8248,#8249,#8250));
#2031=EDGE_LOOP('',(#8251,#8252,#8253,#8254));
#2032=EDGE_LOOP('',(#8255,#8256,#8257,#8258,#8259,#8260,#8261,#8262));
#2033=EDGE_LOOP('',(#8263,#8264,#8265,#8266));
#2034=EDGE_LOOP('',(#8267));
#2035=EDGE_LOOP('',(#8268,#8269,#8270,#8271,#8272,#8273,#8274,#8275));
#2036=EDGE_LOOP('',(#8276,#8277,#8278,#8279));
#2037=EDGE_LOOP('',(#8280,#8281,#8282,#8283,#8284,#8285,#8286,#8287));
#2038=EDGE_LOOP('',(#8288,#8289,#8290,#8291));
#2039=EDGE_LOOP('',(#8292,#8293,#8294,#8295,#8296,#8297,#8298,#8299));
#2040=EDGE_LOOP('',(#8300,#8301,#8302,#8303));
#2041=EDGE_LOOP('',(#8304,#8305,#8306,#8307));
#2042=EDGE_LOOP('',(#8308,#8309,#8310,#8311));
#2043=EDGE_LOOP('',(#8312,#8313,#8314,#8315));
#2044=EDGE_LOOP('',(#8316,#8317,#8318,#8319));
#2045=EDGE_LOOP('',(#8320,#8321,#8322,#8323,#8324,#8325));
#2046=EDGE_LOOP('',(#8326,#8327,#8328,#8329,#8330));
#2047=EDGE_LOOP('',(#8331,#8332,#8333,#8334));
#2048=EDGE_LOOP('',(#8335,#8336,#8337,#8338,#8339,#8340,#8341));
#2049=EDGE_LOOP('',(#8342,#8343,#8344,#8345,#8346,#8347,#8348,#8349));
#2050=EDGE_LOOP('',(#8350));
#2051=EDGE_LOOP('',(#8351));
#2052=EDGE_LOOP('',(#8352));
#2053=EDGE_LOOP('',(#8353));
#2054=EDGE_LOOP('',(#8354));
#2055=EDGE_LOOP('',(#8355));
#2056=EDGE_LOOP('',(#8356,#8357,#8358,#8359));
#2057=EDGE_LOOP('',(#8360,#8361,#8362,#8363));
#2058=EDGE_LOOP('',(#8364,#8365,#8366,#8367));
#2059=EDGE_LOOP('',(#8368,#8369,#8370,#8371));
#2060=EDGE_LOOP('',(#8372,#8373,#8374,#8375,#8376,#8377,#8378,#8379,#8380,
#8381,#8382,#8383,#8384,#8385,#8386,#8387,#8388,#8389,#8390));
#2061=EDGE_LOOP('',(#8391));
#2062=EDGE_LOOP('',(#8392));
#2063=EDGE_LOOP('',(#8393));
#2064=EDGE_LOOP('',(#8394));
#2065=EDGE_LOOP('',(#8395));
#2066=EDGE_LOOP('',(#8396,#8397,#8398,#8399));
#2067=EDGE_LOOP('',(#8400));
#2068=EDGE_LOOP('',(#8401,#8402,#8403,#8404,#8405));
#2069=EDGE_LOOP('',(#8406,#8407,#8408,#8409,#8410,#8411,#8412,#8413));
#2070=EDGE_LOOP('',(#8414,#8415,#8416,#8417,#8418,#8419,#8420,#8421));
#2071=EDGE_LOOP('',(#8422,#8423,#8424,#8425,#8426));
#2072=EDGE_LOOP('',(#8427));
#2073=EDGE_LOOP('',(#8428,#8429,#8430,#8431));
#2074=EDGE_LOOP('',(#8432,#8433,#8434,#8435));
#2075=EDGE_LOOP('',(#8436,#8437,#8438,#8439));
#2076=EDGE_LOOP('',(#8440,#8441,#8442,#8443));
#2077=EDGE_LOOP('',(#8444,#8445,#8446,#8447));
#2078=EDGE_LOOP('',(#8448,#8449,#8450,#8451,#8452,#8453,#8454));
#2079=EDGE_LOOP('',(#8455,#8456,#8457,#8458));
#2080=EDGE_LOOP('',(#8459,#8460,#8461,#8462,#8463));
#2081=EDGE_LOOP('',(#8464,#8465,#8466,#8467,#8468,#8469,#8470,#8471));
#2082=EDGE_LOOP('',(#8472));
#2083=EDGE_LOOP('',(#8473));
#2084=EDGE_LOOP('',(#8474));
#2085=EDGE_LOOP('',(#8475));
#2086=EDGE_LOOP('',(#8476));
#2087=EDGE_LOOP('',(#8477));
#2088=EDGE_LOOP('',(#8478,#8479,#8480,#8481));
#2089=EDGE_LOOP('',(#8482,#8483,#8484,#8485));
#2090=EDGE_LOOP('',(#8486,#8487,#8488,#8489));
#2091=EDGE_LOOP('',(#8490,#8491,#8492,#8493));
#2092=EDGE_LOOP('',(#8494,#8495,#8496,#8497,#8498,#8499,#8500,#8501));
#2093=EDGE_LOOP('',(#8502,#8503,#8504,#8505,#8506,#8507,#8508,#8509));
#2094=EDGE_LOOP('',(#8510,#8511,#8512,#8513));
#2095=EDGE_LOOP('',(#8514,#8515,#8516,#8517));
#2096=EDGE_LOOP('',(#8518,#8519,#8520,#8521));
#2097=EDGE_LOOP('',(#8522,#8523,#8524,#8525));
#2098=EDGE_LOOP('',(#8526,#8527,#8528,#8529,#8530));
#2099=EDGE_LOOP('',(#8531,#8532,#8533,#8534,#8535));
#2100=EDGE_LOOP('',(#8536,#8537,#8538,#8539));
#2101=EDGE_LOOP('',(#8540,#8541,#8542,#8543,#8544));
#2102=EDGE_LOOP('',(#8545,#8546,#8547,#8548,#8549));
#2103=EDGE_LOOP('',(#8550,#8551,#8552,#8553));
#2104=EDGE_LOOP('',(#8554,#8555,#8556));
#2105=EDGE_LOOP('',(#8557,#8558,#8559));
#2106=EDGE_LOOP('',(#8560,#8561,#8562,#8563));
#2107=EDGE_LOOP('',(#8564,#8565,#8566,#8567));
#2108=EDGE_LOOP('',(#8568,#8569,#8570,#8571));
#2109=EDGE_LOOP('',(#8572,#8573,#8574,#8575,#8576));
#2110=EDGE_LOOP('',(#8577,#8578,#8579,#8580,#8581));
#2111=EDGE_LOOP('',(#8582,#8583,#8584,#8585,#8586,#8587));
#2112=EDGE_LOOP('',(#8588,#8589,#8590,#8591,#8592,#8593));
#2113=EDGE_LOOP('',(#8594,#8595,#8596,#8597));
#2114=EDGE_LOOP('',(#8598,#8599,#8600,#8601));
#2115=EDGE_LOOP('',(#8602,#8603,#8604,#8605,#8606));
#2116=EDGE_LOOP('',(#8607,#8608,#8609,#8610,#8611));
#2117=EDGE_LOOP('',(#8612,#8613,#8614,#8615));
#2118=EDGE_LOOP('',(#8616,#8617,#8618,#8619));
#2119=EDGE_LOOP('',(#8620,#8621,#8622,#8623));
#2120=EDGE_LOOP('',(#8624,#8625,#8626,#8627));
#2121=EDGE_LOOP('',(#8628,#8629,#8630,#8631));
#2122=EDGE_LOOP('',(#8632,#8633,#8634,#8635));
#2123=EDGE_LOOP('',(#8636,#8637,#8638,#8639));
#2124=EDGE_LOOP('',(#8640,#8641,#8642,#8643));
#2125=EDGE_LOOP('',(#8644,#8645,#8646,#8647));
#2126=EDGE_LOOP('',(#8648,#8649,#8650,#8651,#8652,#8653));
#2127=EDGE_LOOP('',(#8654,#8655,#8656,#8657,#8658,#8659));
#2128=EDGE_LOOP('',(#8660,#8661,#8662,#8663,#8664,#8665));
#2129=EDGE_LOOP('',(#8666,#8667,#8668,#8669,#8670,#8671));
#2130=EDGE_LOOP('',(#8672,#8673,#8674,#8675,#8676));
#2131=EDGE_LOOP('',(#8677,#8678,#8679,#8680,#8681));
#2132=EDGE_LOOP('',(#8682,#8683,#8684,#8685,#8686));
#2133=EDGE_LOOP('',(#8687,#8688,#8689,#8690,#8691,#8692));
#2134=EDGE_LOOP('',(#8693,#8694,#8695,#8696,#8697,#8698));
#2754=LINE('',#17426,#3574);
#2755=LINE('',#17432,#3575);
#2756=LINE('',#17438,#3576);
#2757=LINE('',#17444,#3577);
#2758=LINE('',#17450,#3578);
#2759=LINE('',#17456,#3579);
#2760=LINE('',#17463,#3580);
#2761=LINE('',#17479,#3581);
#2762=LINE('',#17570,#3582);
#2763=LINE('',#17576,#3583);
#2764=LINE('',#17591,#3584);
#2765=LINE('',#17594,#3585);
#2766=LINE('',#17596,#3586);
#2767=LINE('',#17610,#3587);
#2768=LINE('',#17613,#3588);
#2769=LINE('',#17616,#3589);
#2770=LINE('',#17619,#3590);
#2771=LINE('',#17625,#3591);
#2772=LINE('',#17631,#3592);
#2773=LINE('',#17637,#3593);
#2774=LINE('',#17640,#3594);
#2775=LINE('',#17642,#3595);
#2776=LINE('',#17656,#3596);
#2777=LINE('',#17659,#3597);
#2778=LINE('',#17665,#3598);
#2779=LINE('',#17671,#3599);
#2780=LINE('',#17677,#3600);
#2781=LINE('',#17680,#3601);
#2782=LINE('',#17685,#3602);
#2783=LINE('',#17689,#3603);
#2784=LINE('',#17692,#3604);
#2785=LINE('',#17697,#3605);
#2786=LINE('',#17702,#3606);
#2787=LINE('',#17704,#3607);
#2788=LINE('',#17706,#3608);
#2789=LINE('',#17709,#3609);
#2790=LINE('',#17713,#3610);
#2791=LINE('',#17715,#3611);
#2792=LINE('',#17717,#3612);
#2793=LINE('',#17718,#3613);
#2794=LINE('',#17721,#3614);
#2795=LINE('',#17723,#3615);
#2796=LINE('',#17725,#3616);
#2797=LINE('',#17726,#3617);
#2798=LINE('',#17730,#3618);
#2799=LINE('',#17732,#3619);
#2800=LINE('',#17734,#3620);
#2801=LINE('',#17736,#3621);
#2802=LINE('',#17741,#3622);
#2803=LINE('',#17743,#3623);
#2804=LINE('',#17745,#3624);
#2805=LINE('',#17746,#3625);
#2806=LINE('',#17750,#3626);
#2807=LINE('',#17752,#3627);
#2808=LINE('',#17754,#3628);
#2809=LINE('',#17757,#3629);
#2810=LINE('',#17763,#3630);
#2811=LINE('',#17769,#3631);
#2812=LINE('',#17781,#3632);
#2813=LINE('',#17783,#3633);
#2814=LINE('',#17785,#3634);
#2815=LINE('',#17789,#3635);
#2816=LINE('',#17794,#3636);
#2817=LINE('',#17796,#3637);
#2818=LINE('',#17798,#3638);
#2819=LINE('',#17799,#3639);
#2820=LINE('',#17802,#3640);
#2821=LINE('',#17804,#3641);
#2822=LINE('',#17805,#3642);
#2823=LINE('',#17807,#3643);
#2824=LINE('',#17809,#3644);
#2825=LINE('',#17810,#3645);
#2826=LINE('',#17815,#3646);
#2827=LINE('',#17820,#3647);
#2828=LINE('',#17825,#3648);
#2829=LINE('',#17827,#3649);
#2830=LINE('',#17828,#3650);
#2831=LINE('',#17831,#3651);
#2832=LINE('',#17833,#3652);
#2833=LINE('',#17834,#3653);
#2834=LINE('',#17837,#3654);
#2835=LINE('',#17838,#3655);
#2836=LINE('',#17842,#3656);
#2837=LINE('',#17843,#3657);
#2838=LINE('',#17849,#3658);
#2839=LINE('',#17854,#3659);
#2840=LINE('',#17857,#3660);
#2841=LINE('',#17859,#3661);
#2842=LINE('',#17860,#3662);
#2843=LINE('',#17862,#3663);
#2844=LINE('',#17866,#3664);
#2845=LINE('',#17870,#3665);
#2846=LINE('',#17872,#3666);
#2847=LINE('',#17877,#3667);
#2848=LINE('',#17881,#3668);
#2849=LINE('',#17886,#3669);
#2850=LINE('',#17890,#3670);
#2851=LINE('',#17894,#3671);
#2852=LINE('',#17901,#3672);
#2853=LINE('',#17905,#3673);
#2854=LINE('',#17910,#3674);
#2855=LINE('',#17911,#3675);
#2856=LINE('',#17912,#3676);
#2857=LINE('',#17916,#3677);
#2858=LINE('',#17918,#3678);
#2859=LINE('',#17920,#3679);
#2860=LINE('',#17921,#3680);
#2861=LINE('',#17926,#3681);
#2862=LINE('',#17932,#3682);
#2863=LINE('',#17936,#3683);
#2864=LINE('',#17940,#3684);
#2865=LINE('',#17944,#3685);
#2866=LINE('',#17948,#3686);
#2867=LINE('',#17950,#3687);
#2868=LINE('',#17955,#3688);
#2869=LINE('',#17958,#3689);
#2870=LINE('',#17962,#3690);
#2871=LINE('',#17965,#3691);
#2872=LINE('',#17966,#3692);
#2873=LINE('',#17968,#3693);
#2874=LINE('',#17969,#3694);
#2875=LINE('',#17971,#3695);
#2876=LINE('',#17972,#3696);
#2877=LINE('',#17974,#3697);
#2878=LINE('',#17975,#3698);
#2879=LINE('',#17977,#3699);
#2880=LINE('',#17978,#3700);
#2881=LINE('',#17983,#3701);
#2882=LINE('',#17984,#3702);
#2883=LINE('',#17986,#3703);
#2884=LINE('',#17990,#3704);
#2885=LINE('',#17994,#3705);
#2886=LINE('',#17996,#3706);
#2887=LINE('',#18000,#3707);
#2888=LINE('',#18006,#3708);
#2889=LINE('',#18007,#3709);
#2890=LINE('',#18011,#3710);
#2891=LINE('',#18012,#3711);
#2892=LINE('',#18013,#3712);
#2893=LINE('',#18016,#3713);
#2894=LINE('',#18020,#3714);
#2895=LINE('',#18023,#3715);
#2896=LINE('',#18027,#3716);
#2897=LINE('',#18031,#3717);
#2898=LINE('',#18032,#3718);
#2899=LINE('',#18036,#3719);
#2900=LINE('',#18038,#3720);
#2901=LINE('',#18039,#3721);
#2902=LINE('',#18043,#3722);
#2903=LINE('',#18047,#3723);
#2904=LINE('',#18048,#3724);
#2905=LINE('',#18052,#3725);
#2906=LINE('',#18054,#3726);
#2907=LINE('',#18056,#3727);
#2908=LINE('',#18057,#3728);
#2909=LINE('',#18060,#3729);
#2910=LINE('',#18077,#3730);
#2911=LINE('',#18079,#3731);
#2912=LINE('',#18081,#3732);
#2913=LINE('',#18082,#3733);
#2914=LINE('',#18086,#3734);
#2915=LINE('',#18088,#3735);
#2916=LINE('',#18090,#3736);
#2917=LINE('',#18095,#3737);
#2918=LINE('',#18097,#3738);
#2919=LINE('',#18101,#3739);
#2920=LINE('',#18103,#3740);
#2921=LINE('',#18106,#3741);
#2922=LINE('',#18109,#3742);
#2923=LINE('',#18110,#3743);
#2924=LINE('',#18115,#3744);
#2925=LINE('',#18116,#3745);
#2926=LINE('',#18124,#3746);
#2927=LINE('',#18126,#3747);
#2928=LINE('',#18127,#3748);
#2929=LINE('',#18130,#3749);
#2930=LINE('',#18131,#3750);
#2931=LINE('',#18134,#3751);
#2932=LINE('',#18135,#3752);
#2933=LINE('',#18139,#3753);
#2934=LINE('',#18140,#3754);
#2935=LINE('',#18141,#3755);
#2936=LINE('',#18146,#3756);
#2937=LINE('',#18152,#3757);
#2938=LINE('',#18157,#3758);
#2939=LINE('',#18158,#3759);
#2940=LINE('',#18161,#3760);
#2941=LINE('',#18163,#3761);
#2942=LINE('',#18165,#3762);
#2943=LINE('',#18170,#3763);
#2944=LINE('',#18171,#3764);
#2945=LINE('',#18174,#3765);
#2946=LINE('',#18176,#3766);
#2947=LINE('',#18177,#3767);
#2948=LINE('',#18187,#3768);
#2949=LINE('',#18189,#3769);
#2950=LINE('',#18190,#3770);
#2951=LINE('',#18193,#3771);
#2952=LINE('',#18194,#3772);
#2953=LINE('',#18199,#3773);
#2954=LINE('',#18201,#3774);
#2955=LINE('',#18202,#3775);
#2956=LINE('',#18205,#3776);
#2957=LINE('',#18206,#3777);
#2958=LINE('',#18209,#3778);
#2959=LINE('',#18221,#3779);
#2960=LINE('',#18223,#3780);
#2961=LINE('',#18225,#3781);
#2962=LINE('',#18226,#3782);
#2963=LINE('',#18232,#3783);
#2964=LINE('',#18234,#3784);
#2965=LINE('',#18236,#3785);
#2966=LINE('',#18237,#3786);
#2967=LINE('',#18242,#3787);
#2968=LINE('',#18247,#3788);
#2969=LINE('',#18252,#3789);
#2970=LINE('',#18257,#3790);
#3574=VECTOR('',#13740,13.);
#3575=VECTOR('',#13747,12.4000000000001);
#3576=VECTOR('',#13754,13.);
#3577=VECTOR('',#13761,16.);
#3578=VECTOR('',#13768,12.4000000000001);
#3579=VECTOR('',#13775,15.4);
#3580=VECTOR('',#13782,1000.);
#3581=VECTOR('',#13785,1000.);
#3582=VECTOR('',#13894,1000.);
#3583=VECTOR('',#13899,1000.);
#3584=VECTOR('',#13916,6.00000000000001);
#3585=VECTOR('',#13921,13.);
#3586=VECTOR('',#13924,13.);
#3587=VECTOR('',#13927,16.);
#3588=VECTOR('',#13930,1000.);
#3589=VECTOR('',#13933,1000.);
#3590=VECTOR('',#13936,9.50000000000001);
#3591=VECTOR('',#13943,5.99999999999999);
#3592=VECTOR('',#13950,8.00000000000001);
#3593=VECTOR('',#13957,7.99999999999999);
#3594=VECTOR('',#13962,13.);
#3595=VECTOR('',#13965,13.);
#3596=VECTOR('',#13968,16.);
#3597=VECTOR('',#13971,9.50000000000001);
#3598=VECTOR('',#13978,5.99999999999999);
#3599=VECTOR('',#13985,8.00000000000001);
#3600=VECTOR('',#13992,7.99999999999999);
#3601=VECTOR('',#13997,9.50000000000001);
#3602=VECTOR('',#14002,5.);
#3603=VECTOR('',#14007,1000.);
#3604=VECTOR('',#14010,1000.);
#3605=VECTOR('',#14015,5.);
#3606=VECTOR('',#14020,1000.);
#3607=VECTOR('',#14021,1000.);
#3608=VECTOR('',#14022,1000.);
#3609=VECTOR('',#14025,1000.);
#3610=VECTOR('',#14028,1000.);
#3611=VECTOR('',#14029,1000.);
#3612=VECTOR('',#14030,1000.);
#3613=VECTOR('',#14031,1000.);
#3614=VECTOR('',#14034,1000.);
#3615=VECTOR('',#14035,1000.);
#3616=VECTOR('',#14036,1000.);
#3617=VECTOR('',#14037,1000.);
#3618=VECTOR('',#14040,1000.);
#3619=VECTOR('',#14041,1000.);
#3620=VECTOR('',#14042,1000.);
#3621=VECTOR('',#14043,1000.);
#3622=VECTOR('',#14048,1000.);
#3623=VECTOR('',#14049,1000.);
#3624=VECTOR('',#14050,1000.);
#3625=VECTOR('',#14051,1000.);
#3626=VECTOR('',#14054,1000.);
#3627=VECTOR('',#14055,1000.);
#3628=VECTOR('',#14056,1000.);
#3629=VECTOR('',#14059,1000.);
#3630=VECTOR('',#14064,1000.);
#3631=VECTOR('',#14071,1000.);
#3632=VECTOR('',#14076,1000.);
#3633=VECTOR('',#14077,1000.);
#3634=VECTOR('',#14078,1000.);
#3635=VECTOR('',#14081,1000.);
#3636=VECTOR('',#14086,1000.);
#3637=VECTOR('',#14087,1000.);
#3638=VECTOR('',#14088,1000.);
#3639=VECTOR('',#14089,1000.);
#3640=VECTOR('',#14092,1000.);
#3641=VECTOR('',#14093,1000.);
#3642=VECTOR('',#14094,1000.);
#3643=VECTOR('',#14095,1000.);
#3644=VECTOR('',#14096,1000.);
#3645=VECTOR('',#14097,1000.);
#3646=VECTOR('',#14102,1000.);
#3647=VECTOR('',#14107,1000.);
#3648=VECTOR('',#14114,1000.);
#3649=VECTOR('',#14115,1000.);
#3650=VECTOR('',#14116,1000.);
#3651=VECTOR('',#14119,1000.);
#3652=VECTOR('',#14120,1000.);
#3653=VECTOR('',#14121,1000.);
#3654=VECTOR('',#14124,1000.);
#3655=VECTOR('',#14125,1000.);
#3656=VECTOR('',#14130,1000.);
#3657=VECTOR('',#14131,1000.);
#3658=VECTOR('',#14138,1000.);
#3659=VECTOR('',#14143,1000.);
#3660=VECTOR('',#14146,1000.);
#3661=VECTOR('',#14147,1000.);
#3662=VECTOR('',#14148,1000.);
#3663=VECTOR('',#14149,1000.);
#3664=VECTOR('',#14152,1000.);
#3665=VECTOR('',#14155,1000.);
#3666=VECTOR('',#14158,1000.);
#3667=VECTOR('',#14163,1000.);
#3668=VECTOR('',#14166,1000.);
#3669=VECTOR('',#14171,1000.);
#3670=VECTOR('',#14174,1000.);
#3671=VECTOR('',#14177,1000.);
#3672=VECTOR('',#14184,1000.);
#3673=VECTOR('',#14187,1000.);
#3674=VECTOR('',#14192,1000.);
#3675=VECTOR('',#14193,1000.);
#3676=VECTOR('',#14194,1000.);
#3677=VECTOR('',#14197,1000.);
#3678=VECTOR('',#14198,1000.);
#3679=VECTOR('',#14199,1000.);
#3680=VECTOR('',#14200,1000.);
#3681=VECTOR('',#14205,1000.);
#3682=VECTOR('',#14212,1000.);
#3683=VECTOR('',#14215,1000.);
#3684=VECTOR('',#14218,1000.);
#3685=VECTOR('',#14221,1000.);
#3686=VECTOR('',#14224,1000.);
#3687=VECTOR('',#14225,1000.);
#3688=VECTOR('',#14230,1000.);
#3689=VECTOR('',#14233,1000.);
#3690=VECTOR('',#14236,1000.);
#3691=VECTOR('',#14239,1000.);
#3692=VECTOR('',#14240,1000.);
#3693=VECTOR('',#14243,1000.);
#3694=VECTOR('',#14244,1000.);
#3695=VECTOR('',#14247,1000.);
#3696=VECTOR('',#14248,1000.);
#3697=VECTOR('',#14251,1000.);
#3698=VECTOR('',#14252,1000.);
#3699=VECTOR('',#14255,1000.);
#3700=VECTOR('',#14256,1000.);
#3701=VECTOR('',#14261,1000.);
#3702=VECTOR('',#14262,1000.);
#3703=VECTOR('',#14265,1000.);
#3704=VECTOR('',#14268,1000.);
#3705=VECTOR('',#14275,1000.);
#3706=VECTOR('',#14276,1000.);
#3707=VECTOR('',#14279,1000.);
#3708=VECTOR('',#14286,1000.);
#3709=VECTOR('',#14287,1000.);
#3710=VECTOR('',#14290,1000.);
#3711=VECTOR('',#14291,1000.);
#3712=VECTOR('',#14292,1000.);
#3713=VECTOR('',#14295,1000.);
#3714=VECTOR('',#14300,1000.);
#3715=VECTOR('',#14303,1000.);
#3716=VECTOR('',#14306,1000.);
#3717=VECTOR('',#14309,1000.);
#3718=VECTOR('',#14310,1000.);
#3719=VECTOR('',#14315,1000.);
#3720=VECTOR('',#14316,1000.);
#3721=VECTOR('',#14317,1000.);
#3722=VECTOR('',#14322,1000.);
#3723=VECTOR('',#14327,1000.);
#3724=VECTOR('',#14328,1000.);
#3725=VECTOR('',#14331,1000.);
#3726=VECTOR('',#14332,1000.);
#3727=VECTOR('',#14333,1000.);
#3728=VECTOR('',#14334,1000.);
#3729=VECTOR('',#14337,1000.);
#3730=VECTOR('',#14352,1000.);
#3731=VECTOR('',#14353,1000.);
#3732=VECTOR('',#14354,1000.);
#3733=VECTOR('',#14355,1000.);
#3734=VECTOR('',#14358,1000.);
#3735=VECTOR('',#14359,1000.);
#3736=VECTOR('',#14360,1000.);
#3737=VECTOR('',#14367,1000.);
#3738=VECTOR('',#14370,1000.);
#3739=VECTOR('',#14373,1000.);
#3740=VECTOR('',#14374,1000.);
#3741=VECTOR('',#14377,1000.);
#3742=VECTOR('',#14380,1000.);
#3743=VECTOR('',#14381,1000.);
#3744=VECTOR('',#14388,1000.);
#3745=VECTOR('',#14389,1000.);
#3746=VECTOR('',#14402,1000.);
#3747=VECTOR('',#14403,1000.);
#3748=VECTOR('',#14404,1000.);
#3749=VECTOR('',#14407,1000.);
#3750=VECTOR('',#14408,1000.);
#3751=VECTOR('',#14411,1000.);
#3752=VECTOR('',#14412,1000.);
#3753=VECTOR('',#14415,1000.);
#3754=VECTOR('',#14416,1000.);
#3755=VECTOR('',#14417,1000.);
#3756=VECTOR('',#14422,1000.);
#3757=VECTOR('',#14431,1000.);
#3758=VECTOR('',#14440,1000.);
#3759=VECTOR('',#14441,1000.);
#3760=VECTOR('',#14444,1000.);
#3761=VECTOR('',#14445,1000.);
#3762=VECTOR('',#14446,1000.);
#3763=VECTOR('',#14453,1000.);
#3764=VECTOR('',#14454,1000.);
#3765=VECTOR('',#14459,1000.);
#3766=VECTOR('',#14462,1000.);
#3767=VECTOR('',#14463,1000.);
#3768=VECTOR('',#14476,1000.);
#3769=VECTOR('',#14477,1000.);
#3770=VECTOR('',#14478,1000.);
#3771=VECTOR('',#14481,1000.);
#3772=VECTOR('',#14482,1000.);
#3773=VECTOR('',#14489,1000.);
#3774=VECTOR('',#14490,1000.);
#3775=VECTOR('',#14491,1000.);
#3776=VECTOR('',#14494,1000.);
#3777=VECTOR('',#14495,1000.);
#3778=VECTOR('',#14500,1000.);
#3779=VECTOR('',#14519,1000.);
#3780=VECTOR('',#14520,1000.);
#3781=VECTOR('',#14521,1000.);
#3782=VECTOR('',#14522,1000.);
#3783=VECTOR('',#14529,1000.);
#3784=VECTOR('',#14530,1000.);
#3785=VECTOR('',#14531,1000.);
#3786=VECTOR('',#14532,1000.);
#3787=VECTOR('',#14537,1000.);
#3788=VECTOR('',#14542,1000.);
#3789=VECTOR('',#14547,1000.);
#3790=VECTOR('',#14552,1000.);
#4394=CIRCLE('',#12301,13.);
#4395=CIRCLE('',#12302,12.4);
#4396=CIRCLE('',#12304,13.);
#4397=CIRCLE('',#12305,12.4000000000001);
#4398=CIRCLE('',#12307,13.);
#4399=CIRCLE('',#12308,12.4);
#4400=CIRCLE('',#12310,16.);
#4401=CIRCLE('',#12311,15.3999999999999);
#4402=CIRCLE('',#12313,13.);
#4403=CIRCLE('',#12314,12.4000000000001);
#4404=CIRCLE('',#12316,16.);
#4405=CIRCLE('',#12317,15.4);
#4406=CIRCLE('',#12319,4.5);
#4407=CIRCLE('',#12320,4.5);
#4408=CIRCLE('',#12322,24.);
#4409=CIRCLE('',#12323,6.00000000000001);
#4410=CIRCLE('',#12324,30.);
#4411=CIRCLE('',#12325,6.00000000000001);
#4412=CIRCLE('',#12327,18.);
#4413=CIRCLE('',#12328,2.);
#4414=CIRCLE('',#12329,16.);
#4415=CIRCLE('',#12331,15.);
#4416=CIRCLE('',#12332,2.);
#4417=CIRCLE('',#12333,13.);
#4418=CIRCLE('',#12335,15.);
#4419=CIRCLE('',#12336,2.);
#4420=CIRCLE('',#12337,13.);
#4421=CIRCLE('',#12339,18.);
#4422=CIRCLE('',#12340,2.);
#4423=CIRCLE('',#12341,16.);
#4424=CIRCLE('',#12343,15.);
#4425=CIRCLE('',#12344,2.);
#4426=CIRCLE('',#12345,13.);
#4427=CIRCLE('',#12346,13.);
#4428=CIRCLE('',#12347,2.);
#4429=CIRCLE('',#12349,15.);
#4430=CIRCLE('',#12350,2.);
#4431=CIRCLE('',#12351,13.);
#4432=CIRCLE('',#12352,13.);
#4433=CIRCLE('',#12353,1.99999999999999);
#4434=CIRCLE('',#12355,11.5);
#4435=CIRCLE('',#12356,2.);
#4436=CIRCLE('',#12357,9.50000000000001);
#4437=CIRCLE('',#12358,9.50000000000001);
#4438=CIRCLE('',#12360,11.5);
#4439=CIRCLE('',#12361,2.);
#4440=CIRCLE('',#12362,9.50000000000001);
#4441=CIRCLE('',#12364,9.50000000000001);
#4442=CIRCLE('',#12365,9.50000000000001);
#4443=CIRCLE('',#12366,2.);
#4444=CIRCLE('',#12367,11.5);
#4445=CIRCLE('',#12369,9.50000000000001);
#4446=CIRCLE('',#12370,9.50000000000001);
#4447=CIRCLE('',#12371,2.);
#4448=CIRCLE('',#12372,11.5);
#4449=CIRCLE('',#12374,4.);
#4450=CIRCLE('',#12375,4.);
#4451=CIRCLE('',#12377,4.);
#4452=CIRCLE('',#12379,23.);
#4453=CIRCLE('',#12380,4.);
#4454=CIRCLE('',#12381,27.);
#4455=CIRCLE('',#12382,4.);
#4456=CIRCLE('',#12384,6.00000000000001);
#4457=CIRCLE('',#12385,6.00000000000001);
#4458=CIRCLE('',#12392,9.50000000000001);
#4459=CIRCLE('',#12394,5.99999999999999);
#4460=CIRCLE('',#12395,5.99999999999999);
#4461=CIRCLE('',#12397,8.00000000000001);
#4462=CIRCLE('',#12398,8.00000000000001);
#4463=CIRCLE('',#12400,7.99999999999999);
#4464=CIRCLE('',#12401,7.99999999999999);
#4465=CIRCLE('',#12406,9.50000000000001);
#4466=CIRCLE('',#12408,5.99999999999999);
#4467=CIRCLE('',#12409,5.99999999999999);
#4468=CIRCLE('',#12411,8.00000000000001);
#4469=CIRCLE('',#12412,8.00000000000001);
#4470=CIRCLE('',#12414,7.99999999999999);
#4471=CIRCLE('',#12415,7.99999999999999);
#4472=CIRCLE('',#12418,5.);
#4473=CIRCLE('',#12419,5.);
#4474=CIRCLE('',#12423,5.);
#4475=CIRCLE('',#12424,5.);
#4476=CIRCLE('',#12426,4.);
#4477=CIRCLE('',#12430,4.);
#4478=CIRCLE('',#12433,4.);
#4479=CIRCLE('',#12436,100.);
#4480=CIRCLE('',#12437,100.);
#4481=CIRCLE('',#12438,100.);
#4482=CIRCLE('',#12439,100.);
#4483=CIRCLE('',#12441,53.);
#4484=CIRCLE('',#12442,53.);
#4485=CIRCLE('',#12446,10.);
#4486=CIRCLE('',#12447,10.);
#4487=CIRCLE('',#12454,2.);
#4488=CIRCLE('',#12458,2.);
#4489=CIRCLE('',#12459,2.);
#4490=CIRCLE('',#12460,15.);
#4491=CIRCLE('',#12461,15.);
#4492=CIRCLE('',#12462,15.);
#4493=CIRCLE('',#12463,15.);
#4494=CIRCLE('',#12464,6.00000000000001);
#4495=CIRCLE('',#12467,2.);
#4496=CIRCLE('',#12468,2.);
#4497=CIRCLE('',#12469,15.);
#4498=CIRCLE('',#12470,15.);
#4499=CIRCLE('',#12471,4.5);
#4500=CIRCLE('',#12472,4.5);
#4501=CIRCLE('',#12473,100.);
#4502=CIRCLE('',#12474,100.);
#4503=CIRCLE('',#12475,15.);
#4504=CIRCLE('',#12476,15.);
#4505=CIRCLE('',#12480,10.);
#4506=CIRCLE('',#12481,10.);
#4507=CIRCLE('',#12483,2.);
#4508=CIRCLE('',#12484,2.);
#4509=CIRCLE('',#12485,15.);
#4510=CIRCLE('',#12486,15.);
#4511=CIRCLE('',#12487,100.);
#4512=CIRCLE('',#12488,4.5);
#4513=CIRCLE('',#12489,15.);
#4514=CIRCLE('',#12490,15.);
#4515=CIRCLE('',#12491,6.00000000000001);
#4516=CIRCLE('',#12499,2.);
#4517=CIRCLE('',#12501,30.);
#4518=CIRCLE('',#12507,24.);
#4519=CIRCLE('',#12514,23.);
#4520=CIRCLE('',#12516,2.);
#4521=CIRCLE('',#12518,27.);
#4522=CIRCLE('',#12524,100.);
#4523=CIRCLE('',#12531,53.);
#4524=CIRCLE('',#12532,53.);
#4525=CIRCLE('',#12536,3.99999999999999);
#4526=CIRCLE('',#12541,53.);
#4527=CIRCLE('',#12542,53.);
#4528=CIRCLE('',#12551,2.);
#4529=CIRCLE('',#12552,2.);
#4530=CIRCLE('',#12553,15.);
#4531=CIRCLE('',#12554,15.);
#4532=CIRCLE('',#12555,4.5);
#4533=CIRCLE('',#12556,15.);
#4534=CIRCLE('',#12557,15.);
#4535=CIRCLE('',#12563,2.);
#4536=CIRCLE('',#12572,3.99999999999999);
#4537=CIRCLE('',#12580,53.);
#4538=CIRCLE('',#12581,53.);
#4539=CIRCLE('',#12586,4.);
#4540=CIRCLE('',#12587,4.);
#4541=CIRCLE('',#12590,4.);
#4542=CIRCLE('',#12593,6.50000000000001);
#4543=CIRCLE('',#12594,2.);
#4544=CIRCLE('',#12595,2.);
#4545=CIRCLE('',#12596,6.50000000000001);
#4546=CIRCLE('',#12598,6.50000000000001);
#4547=CIRCLE('',#12599,6.50000000000001);
#4548=CIRCLE('',#12600,2.);
#4549=CIRCLE('',#12601,2.);
#4550=CIRCLE('',#12611,4.);
#4551=CIRCLE('',#12613,4.);
#4552=CIRCLE('',#12615,3.99999999999998);
#4553=CIRCLE('',#12616,3.99999999999998);
#4554=CIRCLE('',#12618,4.);
#4555=CIRCLE('',#12620,4.);
#4556=CIRCLE('',#12622,4.);
#4557=CIRCLE('',#12624,4.);
#4558=CIRCLE('',#12639,6.00000000000001);
#4559=CIRCLE('',#12641,5.99999999999999);
#5035=VERTEX_POINT('',#17423);
#5036=VERTEX_POINT('',#17425);
#5037=VERTEX_POINT('',#17429);
#5038=VERTEX_POINT('',#17431);
#5039=VERTEX_POINT('',#17435);
#5040=VERTEX_POINT('',#17437);
#5041=VERTEX_POINT('',#17441);
#5042=VERTEX_POINT('',#17443);
#5043=VERTEX_POINT('',#17447);
#5044=VERTEX_POINT('',#17449);
#5045=VERTEX_POINT('',#17453);
#5046=VERTEX_POINT('',#17455);
#5047=VERTEX_POINT('',#17459);
#5048=VERTEX_POINT('',#17460);
#5049=VERTEX_POINT('',#17462);
#5050=VERTEX_POINT('',#17464);
#5051=VERTEX_POINT('',#17466);
#5052=VERTEX_POINT('',#17481);
#5053=VERTEX_POINT('',#17482);
#5054=VERTEX_POINT('',#17484);
#5055=VERTEX_POINT('',#17486);
#5056=VERTEX_POINT('',#17490);
#5057=VERTEX_POINT('',#17492);
#5058=VERTEX_POINT('',#17496);
#5059=VERTEX_POINT('',#17498);
#5060=VERTEX_POINT('',#17502);
#5061=VERTEX_POINT('',#17504);
#5062=VERTEX_POINT('',#17508);
#5063=VERTEX_POINT('',#17510);
#5064=VERTEX_POINT('',#17514);
#5065=VERTEX_POINT('',#17515);
#5066=VERTEX_POINT('',#17517);
#5067=VERTEX_POINT('',#17519);
#5068=VERTEX_POINT('',#17521);
#5069=VERTEX_POINT('',#17525);
#5070=VERTEX_POINT('',#17526);
#5071=VERTEX_POINT('',#17528);
#5072=VERTEX_POINT('',#17530);
#5073=VERTEX_POINT('',#17532);
#5074=VERTEX_POINT('',#17536);
#5075=VERTEX_POINT('',#17538);
#5076=VERTEX_POINT('',#17540);
#5077=VERTEX_POINT('',#17544);
#5078=VERTEX_POINT('',#17546);
#5079=VERTEX_POINT('',#17550);
#5080=VERTEX_POINT('',#17551);
#5081=VERTEX_POINT('',#17554);
#5082=VERTEX_POINT('',#17558);
#5083=VERTEX_POINT('',#17559);
#5084=VERTEX_POINT('',#17562);
#5085=VERTEX_POINT('',#17566);
#5086=VERTEX_POINT('',#17567);
#5087=VERTEX_POINT('',#17569);
#5088=VERTEX_POINT('',#17571);
#5089=VERTEX_POINT('',#17573);
#5090=VERTEX_POINT('',#17575);
#5091=VERTEX_POINT('',#17579);
#5092=VERTEX_POINT('',#17580);
#5093=VERTEX_POINT('',#17582);
#5094=VERTEX_POINT('',#17584);
#5095=VERTEX_POINT('',#17588);
#5096=VERTEX_POINT('',#17590);
#5097=VERTEX_POINT('',#17612);
#5098=VERTEX_POINT('',#17614);
#5099=VERTEX_POINT('',#17618);
#5100=VERTEX_POINT('',#17622);
#5101=VERTEX_POINT('',#17624);
#5102=VERTEX_POINT('',#17628);
#5103=VERTEX_POINT('',#17630);
#5104=VERTEX_POINT('',#17634);
#5105=VERTEX_POINT('',#17636);
#5106=VERTEX_POINT('',#17658);
#5107=VERTEX_POINT('',#17662);
#5108=VERTEX_POINT('',#17664);
#5109=VERTEX_POINT('',#17668);
#5110=VERTEX_POINT('',#17670);
#5111=VERTEX_POINT('',#17674);
#5112=VERTEX_POINT('',#17676);
#5113=VERTEX_POINT('',#17682);
#5114=VERTEX_POINT('',#17684);
#5115=VERTEX_POINT('',#17688);
#5116=VERTEX_POINT('',#17690);
#5117=VERTEX_POINT('',#17694);
#5118=VERTEX_POINT('',#17696);
#5119=VERTEX_POINT('',#17700);
#5120=VERTEX_POINT('',#17701);
#5121=VERTEX_POINT('',#17703);
#5122=VERTEX_POINT('',#17705);
#5123=VERTEX_POINT('',#17707);
#5124=VERTEX_POINT('',#17711);
#5125=VERTEX_POINT('',#17712);
#5126=VERTEX_POINT('',#17714);
#5127=VERTEX_POINT('',#17716);
#5128=VERTEX_POINT('',#17720);
#5129=VERTEX_POINT('',#17722);
#5130=VERTEX_POINT('',#17724);
#5131=VERTEX_POINT('',#17728);
#5132=VERTEX_POINT('',#17729);
#5133=VERTEX_POINT('',#17731);
#5134=VERTEX_POINT('',#17733);
#5135=VERTEX_POINT('',#17735);
#5136=VERTEX_POINT('',#17739);
#5137=VERTEX_POINT('',#17740);
#5138=VERTEX_POINT('',#17742);
#5139=VERTEX_POINT('',#17744);
#5140=VERTEX_POINT('',#17748);
#5141=VERTEX_POINT('',#17749);
#5142=VERTEX_POINT('',#17751);
#5143=VERTEX_POINT('',#17753);
#5144=VERTEX_POINT('',#17755);
#5145=VERTEX_POINT('',#17759);
#5146=VERTEX_POINT('',#17760);
#5147=VERTEX_POINT('',#17762);
#5148=VERTEX_POINT('',#17766);
#5149=VERTEX_POINT('',#17768);
#5150=VERTEX_POINT('',#17770);
#5151=VERTEX_POINT('',#17779);
#5152=VERTEX_POINT('',#17780);
#5153=VERTEX_POINT('',#17782);
#5154=VERTEX_POINT('',#17784);
#5155=VERTEX_POINT('',#17786);
#5156=VERTEX_POINT('',#17788);
#5157=VERTEX_POINT('',#17792);
#5158=VERTEX_POINT('',#17793);
#5159=VERTEX_POINT('',#17795);
#5160=VERTEX_POINT('',#17797);
#5161=VERTEX_POINT('',#17801);
#5162=VERTEX_POINT('',#17803);
#5163=VERTEX_POINT('',#17806);
#5164=VERTEX_POINT('',#17808);
#5165=VERTEX_POINT('',#17812);
#5166=VERTEX_POINT('',#17814);
#5167=VERTEX_POINT('',#17818);
#5168=VERTEX_POINT('',#17819);
#5169=VERTEX_POINT('',#17824);
#5170=VERTEX_POINT('',#17826);
#5171=VERTEX_POINT('',#17830);
#5172=VERTEX_POINT('',#17832);
#5173=VERTEX_POINT('',#17836);
#5174=VERTEX_POINT('',#17841);
#5175=VERTEX_POINT('',#17846);
#5176=VERTEX_POINT('',#17848);
#5177=VERTEX_POINT('',#17851);
#5178=VERTEX_POINT('',#17853);
#5179=VERTEX_POINT('',#17855);
#5180=VERTEX_POINT('',#17858);
#5181=VERTEX_POINT('',#17861);
#5182=VERTEX_POINT('',#17863);
#5183=VERTEX_POINT('',#17865);
#5184=VERTEX_POINT('',#17868);
#5185=VERTEX_POINT('',#17869);
#5186=VERTEX_POINT('',#17875);
#5187=VERTEX_POINT('',#17876);
#5188=VERTEX_POINT('',#17878);
#5189=VERTEX_POINT('',#17880);
#5190=VERTEX_POINT('',#17883);
#5191=VERTEX_POINT('',#17885);
#5192=VERTEX_POINT('',#17887);
#5193=VERTEX_POINT('',#17889);
#5194=VERTEX_POINT('',#17891);
#5195=VERTEX_POINT('',#17893);
#5196=VERTEX_POINT('',#17895);
#5197=VERTEX_POINT('',#17898);
#5198=VERTEX_POINT('',#17900);
#5199=VERTEX_POINT('',#17902);
#5200=VERTEX_POINT('',#17904);
#5201=VERTEX_POINT('',#17908);
#5202=VERTEX_POINT('',#17909);
#5203=VERTEX_POINT('',#17914);
#5204=VERTEX_POINT('',#17915);
#5205=VERTEX_POINT('',#17917);
#5206=VERTEX_POINT('',#17919);
#5207=VERTEX_POINT('',#17923);
#5208=VERTEX_POINT('',#17925);
#5209=VERTEX_POINT('',#17929);
#5210=VERTEX_POINT('',#17931);
#5211=VERTEX_POINT('',#17933);
#5212=VERTEX_POINT('',#17935);
#5213=VERTEX_POINT('',#17937);
#5214=VERTEX_POINT('',#17939);
#5215=VERTEX_POINT('',#17941);
#5216=VERTEX_POINT('',#17943);
#5217=VERTEX_POINT('',#17945);
#5218=VERTEX_POINT('',#17947);
#5219=VERTEX_POINT('',#17949);
#5220=VERTEX_POINT('',#17952);
#5221=VERTEX_POINT('',#17954);
#5222=VERTEX_POINT('',#17957);
#5223=VERTEX_POINT('',#17959);
#5224=VERTEX_POINT('',#17961);
#5225=VERTEX_POINT('',#17963);
#5226=VERTEX_POINT('',#17981);
#5227=VERTEX_POINT('',#17982);
#5228=VERTEX_POINT('',#17988);
#5229=VERTEX_POINT('',#17989);
#5230=VERTEX_POINT('',#17995);
#5231=VERTEX_POINT('',#17997);
#5232=VERTEX_POINT('',#17999);
#5233=VERTEX_POINT('',#18003);
#5234=VERTEX_POINT('',#18004);
#5235=VERTEX_POINT('',#18009);
#5236=VERTEX_POINT('',#18010);
#5237=VERTEX_POINT('',#18015);
#5238=VERTEX_POINT('',#18019);
#5239=VERTEX_POINT('',#18021);
#5240=VERTEX_POINT('',#18025);
#5241=VERTEX_POINT('',#18026);
#5242=VERTEX_POINT('',#18028);
#5243=VERTEX_POINT('',#18030);
#5244=VERTEX_POINT('',#18035);
#5245=VERTEX_POINT('',#18037);
#5246=VERTEX_POINT('',#18041);
#5247=VERTEX_POINT('',#18046);
#5248=VERTEX_POINT('',#18050);
#5249=VERTEX_POINT('',#18051);
#5250=VERTEX_POINT('',#18053);
#5251=VERTEX_POINT('',#18055);
#5252=VERTEX_POINT('',#18059);
#5253=VERTEX_POINT('',#18061);
#5254=VERTEX_POINT('',#18075);
#5255=VERTEX_POINT('',#18076);
#5256=VERTEX_POINT('',#18078);
#5257=VERTEX_POINT('',#18080);
#5258=VERTEX_POINT('',#18084);
#5259=VERTEX_POINT('',#18085);
#5260=VERTEX_POINT('',#18087);
#5261=VERTEX_POINT('',#18089);
#5262=VERTEX_POINT('',#18094);
#5263=VERTEX_POINT('',#18099);
#5264=VERTEX_POINT('',#18100);
#5265=VERTEX_POINT('',#18102);
#5266=VERTEX_POINT('',#18104);
#5267=VERTEX_POINT('',#18108);
#5268=VERTEX_POINT('',#18114);
#5269=VERTEX_POINT('',#18123);
#5270=VERTEX_POINT('',#18125);
#5271=VERTEX_POINT('',#18129);
#5272=VERTEX_POINT('',#18133);
#5273=VERTEX_POINT('',#18137);
#5274=VERTEX_POINT('',#18138);
#5275=VERTEX_POINT('',#18143);
#5276=VERTEX_POINT('',#18145);
#5277=VERTEX_POINT('',#18150);
#5278=VERTEX_POINT('',#18160);
#5279=VERTEX_POINT('',#18162);
#5280=VERTEX_POINT('',#18164);
#5281=VERTEX_POINT('',#18169);
#5282=VERTEX_POINT('',#18183);
#5283=VERTEX_POINT('',#18184);
#5284=VERTEX_POINT('',#18186);
#5285=VERTEX_POINT('',#18188);
#5286=VERTEX_POINT('',#18192);
#5287=VERTEX_POINT('',#18198);
#5288=VERTEX_POINT('',#18200);
#5289=VERTEX_POINT('',#18204);
#5290=VERTEX_POINT('',#18219);
#5291=VERTEX_POINT('',#18220);
#5292=VERTEX_POINT('',#18222);
#5293=VERTEX_POINT('',#18224);
#5294=VERTEX_POINT('',#18230);
#5295=VERTEX_POINT('',#18231);
#5296=VERTEX_POINT('',#18233);
#5297=VERTEX_POINT('',#18235);
#5298=VERTEX_POINT('',#18239);
#5299=VERTEX_POINT('',#18241);
#5300=VERTEX_POINT('',#18244);
#5301=VERTEX_POINT('',#18246);
#5302=VERTEX_POINT('',#18250);
#5303=VERTEX_POINT('',#18251);
#5304=VERTEX_POINT('',#18254);
#5305=VERTEX_POINT('',#18256);
#6138=EDGE_CURVE('',#5035,#5035,#4394,.T.);
#6139=EDGE_CURVE('',#5035,#5036,#2754,.T.);
#6140=EDGE_CURVE('',#5036,#5036,#4395,.T.);
#6141=EDGE_CURVE('',#5037,#5037,#4396,.T.);
#6142=EDGE_CURVE('',#5037,#5038,#2755,.T.);
#6143=EDGE_CURVE('',#5038,#5038,#4397,.T.);
#6144=EDGE_CURVE('',#5039,#5039,#4398,.T.);
#6145=EDGE_CURVE('',#5039,#5040,#2756,.T.);
#6146=EDGE_CURVE('',#5040,#5040,#4399,.T.);
#6147=EDGE_CURVE('',#5041,#5041,#4400,.T.);
#6148=EDGE_CURVE('',#5041,#5042,#2757,.T.);
#6149=EDGE_CURVE('',#5042,#5042,#4401,.T.);
#6150=EDGE_CURVE('',#5043,#5043,#4402,.T.);
#6151=EDGE_CURVE('',#5043,#5044,#2758,.T.);
#6152=EDGE_CURVE('',#5044,#5044,#4403,.T.);
#6153=EDGE_CURVE('',#5045,#5045,#4404,.T.);
#6154=EDGE_CURVE('',#5045,#5046,#2759,.T.);
#6155=EDGE_CURVE('',#5046,#5046,#4405,.T.);
#6156=EDGE_CURVE('',#5047,#5048,#4406,.T.);
#6157=EDGE_CURVE('',#5049,#5047,#2760,.T.);
#6158=EDGE_CURVE('',#5050,#5049,#4407,.T.);
#6159=EDGE_CURVE('',#5051,#5050,#850,.F.);
#6160=EDGE_CURVE('',#5051,#5048,#2761,.T.);
#6161=EDGE_CURVE('',#5052,#5053,#4408,.T.);
#6162=EDGE_CURVE('',#5054,#5052,#4409,.T.);
#6163=EDGE_CURVE('',#5055,#5054,#4410,.T.);
#6164=EDGE_CURVE('',#5055,#5053,#4411,.T.);
#6165=EDGE_CURVE('',#5056,#5056,#4412,.T.);
#6166=EDGE_CURVE('',#5056,#5057,#4413,.T.);
#6167=EDGE_CURVE('',#5057,#5057,#4414,.T.);
#6168=EDGE_CURVE('',#5058,#5058,#4415,.T.);
#6169=EDGE_CURVE('',#5058,#5059,#4416,.T.);
#6170=EDGE_CURVE('',#5059,#5059,#4417,.T.);
#6171=EDGE_CURVE('',#5060,#5060,#4418,.T.);
#6172=EDGE_CURVE('',#5060,#5061,#4419,.T.);
#6173=EDGE_CURVE('',#5061,#5061,#4420,.T.);
#6174=EDGE_CURVE('',#5062,#5062,#4421,.T.);
#6175=EDGE_CURVE('',#5062,#5063,#4422,.T.);
#6176=EDGE_CURVE('',#5063,#5063,#4423,.T.);
#6177=EDGE_CURVE('',#5064,#5065,#4424,.T.);
#6178=EDGE_CURVE('',#5066,#5064,#4425,.T.);
#6179=EDGE_CURVE('',#5067,#5066,#4426,.T.);
#6180=EDGE_CURVE('',#5068,#5067,#4427,.T.);
#6181=EDGE_CURVE('',#5065,#5068,#4428,.T.);
#6182=EDGE_CURVE('',#5069,#5070,#4429,.T.);
#6183=EDGE_CURVE('',#5071,#5069,#4430,.T.);
#6184=EDGE_CURVE('',#5072,#5071,#4431,.T.);
#6185=EDGE_CURVE('',#5073,#5072,#4432,.T.);
#6186=EDGE_CURVE('',#5070,#5073,#4433,.T.);
#6187=EDGE_CURVE('',#5074,#5074,#4434,.T.);
#6188=EDGE_CURVE('',#5074,#5075,#4435,.T.);
#6189=EDGE_CURVE('',#5076,#5075,#4436,.T.);
#6190=EDGE_CURVE('',#5075,#5076,#4437,.T.);
#6191=EDGE_CURVE('',#5077,#5077,#4438,.T.);
#6192=EDGE_CURVE('',#5077,#5078,#4439,.T.);
#6193=EDGE_CURVE('',#5078,#5078,#4440,.T.);
#6194=EDGE_CURVE('',#5079,#5080,#4441,.T.);
#6195=EDGE_CURVE('',#5080,#5079,#4442,.T.);
#6196=EDGE_CURVE('',#5080,#5081,#4443,.T.);
#6197=EDGE_CURVE('',#5081,#5081,#4444,.T.);
#6198=EDGE_CURVE('',#5082,#5083,#4445,.T.);
#6199=EDGE_CURVE('',#5083,#5082,#4446,.T.);
#6200=EDGE_CURVE('',#5083,#5084,#4447,.T.);
#6201=EDGE_CURVE('',#5084,#5084,#4448,.T.);
#6202=EDGE_CURVE('',#5085,#5086,#4449,.T.);
#6203=EDGE_CURVE('',#5087,#5085,#2762,.T.);
#6204=EDGE_CURVE('',#5088,#5087,#4450,.T.);
#6205=EDGE_CURVE('',#5088,#5089,#747,.T.);
#6206=EDGE_CURVE('',#5090,#5089,#2763,.T.);
#6207=EDGE_CURVE('',#5086,#5090,#4451,.T.);
#6208=EDGE_CURVE('',#5091,#5092,#4452,.T.);
#6209=EDGE_CURVE('',#5091,#5093,#4453,.T.);
#6210=EDGE_CURVE('',#5094,#5093,#4454,.T.);
#6211=EDGE_CURVE('',#5092,#5094,#4455,.T.);
#6212=EDGE_CURVE('',#5095,#5095,#4456,.T.);
#6213=EDGE_CURVE('',#5095,#5096,#2764,.T.);
#6214=EDGE_CURVE('',#5096,#5096,#4457,.T.);
#6215=EDGE_CURVE('',#5061,#5039,#2765,.T.);
#6216=EDGE_CURVE('',#5067,#5035,#2766,.T.);
#6217=EDGE_CURVE('',#5066,#5068,#851,.T.);
#6218=EDGE_CURVE('',#5063,#5041,#2767,.T.);
#6219=EDGE_CURVE('',#5093,#5097,#2768,.T.);
#6220=EDGE_CURVE('',#5098,#5097,#748,.T.);
#6221=EDGE_CURVE('',#5094,#5098,#2769,.T.);
#6222=EDGE_CURVE('',#5082,#5099,#2770,.T.);
#6223=EDGE_CURVE('',#5099,#5099,#4458,.T.);
#6224=EDGE_CURVE('',#5100,#5100,#4459,.T.);
#6225=EDGE_CURVE('',#5100,#5101,#2771,.T.);
#6226=EDGE_CURVE('',#5101,#5101,#4460,.T.);
#6227=EDGE_CURVE('',#5102,#5102,#4461,.T.);
#6228=EDGE_CURVE('',#5102,#5103,#2772,.T.);
#6229=EDGE_CURVE('',#5103,#5103,#4462,.T.);
#6230=EDGE_CURVE('',#5104,#5104,#4463,.T.);
#6231=EDGE_CURVE('',#5104,#5105,#2773,.T.);
#6232=EDGE_CURVE('',#5105,#5105,#4464,.T.);
#6233=EDGE_CURVE('',#5059,#5043,#2774,.T.);
#6234=EDGE_CURVE('',#5072,#5037,#2775,.T.);
#6235=EDGE_CURVE('',#5071,#5073,#852,.T.);
#6236=EDGE_CURVE('',#5057,#5045,#2776,.T.);
#6237=EDGE_CURVE('',#5079,#5106,#2777,.T.);
#6238=EDGE_CURVE('',#5106,#5106,#4465,.T.);
#6239=EDGE_CURVE('',#5107,#5107,#4466,.T.);
#6240=EDGE_CURVE('',#5107,#5108,#2778,.T.);
#6241=EDGE_CURVE('',#5108,#5108,#4467,.T.);
#6242=EDGE_CURVE('',#5109,#5109,#4468,.T.);
#6243=EDGE_CURVE('',#5109,#5110,#2779,.T.);
#6244=EDGE_CURVE('',#5110,#5110,#4469,.T.);
#6245=EDGE_CURVE('',#5111,#5111,#4470,.T.);
#6246=EDGE_CURVE('',#5111,#5112,#2780,.T.);
#6247=EDGE_CURVE('',#5112,#5112,#4471,.T.);
#6248=EDGE_CURVE('',#5078,#5076,#2781,.T.);
#6249=EDGE_CURVE('',#5113,#5113,#4472,.T.);
#6250=EDGE_CURVE('',#5113,#5114,#2782,.T.);
#6251=EDGE_CURVE('',#5114,#5114,#4473,.T.);
#6252=EDGE_CURVE('',#5054,#5115,#2783,.T.);
#6253=EDGE_CURVE('',#5115,#5116,#749,.T.);
#6254=EDGE_CURVE('',#5055,#5116,#2784,.T.);
#6255=EDGE_CURVE('',#5117,#5117,#4474,.T.);
#6256=EDGE_CURVE('',#5117,#5118,#2785,.T.);
#6257=EDGE_CURVE('',#5118,#5118,#4475,.T.);
#6258=EDGE_CURVE('',#5119,#5120,#2786,.T.);
#6259=EDGE_CURVE('',#5119,#5121,#2787,.T.);
#6260=EDGE_CURVE('',#5121,#5122,#2788,.T.);
#6261=EDGE_CURVE('',#5122,#5123,#4476,.T.);
#6262=EDGE_CURVE('',#5120,#5123,#2789,.T.);
#6263=EDGE_CURVE('',#5124,#5125,#2790,.T.);
#6264=EDGE_CURVE('',#5125,#5126,#2791,.T.);
#6265=EDGE_CURVE('',#5127,#5126,#2792,.T.);
#6266=EDGE_CURVE('',#5127,#5124,#2793,.T.);
#6267=EDGE_CURVE('',#5090,#5128,#2794,.T.);
#6268=EDGE_CURVE('',#5128,#5129,#2795,.T.);
#6269=EDGE_CURVE('',#5130,#5129,#2796,.T.);
#6270=EDGE_CURVE('',#5086,#5130,#2797,.T.);
#6271=EDGE_CURVE('',#5131,#5132,#2798,.T.);
#6272=EDGE_CURVE('',#5131,#5133,#2799,.T.);
#6273=EDGE_CURVE('',#5133,#5134,#2800,.T.);
#6274=EDGE_CURVE('',#5134,#5135,#2801,.T.);
#6275=EDGE_CURVE('',#5135,#5132,#4477,.T.);
#6276=EDGE_CURVE('',#5136,#5137,#2802,.T.);
#6277=EDGE_CURVE('',#5137,#5138,#2803,.T.);
#6278=EDGE_CURVE('',#5139,#5138,#2804,.T.);
#6279=EDGE_CURVE('',#5139,#5136,#2805,.T.);
#6280=EDGE_CURVE('',#5140,#5141,#2806,.T.);
#6281=EDGE_CURVE('',#5141,#5142,#2807,.T.);
#6282=EDGE_CURVE('',#5143,#5142,#2808,.T.);
#6283=EDGE_CURVE('',#5143,#5144,#4478,.T.);
#6284=EDGE_CURVE('',#5144,#5140,#2809,.T.);
#6285=EDGE_CURVE('',#5145,#5146,#750,.T.);
#6286=EDGE_CURVE('',#5145,#5147,#2810,.T.);
#6287=EDGE_CURVE('',#5065,#5147,#4479,.T.);
#6288=EDGE_CURVE('',#5064,#5065,#4480,.T.);
#6289=EDGE_CURVE('',#5148,#5064,#4481,.T.);
#6290=EDGE_CURVE('',#5149,#5148,#2811,.T.);
#6291=EDGE_CURVE('',#5150,#5149,#4482,.T.);
#6292=EDGE_CURVE('',#5150,#5146,#853,.T.);
#6293=EDGE_CURVE('',#5151,#5152,#2812,.T.);
#6294=EDGE_CURVE('',#5152,#5153,#2813,.T.);
#6295=EDGE_CURVE('',#5153,#5154,#2814,.T.);
#6296=EDGE_CURVE('',#5154,#5155,#4483,.T.);
#6297=EDGE_CURVE('',#5155,#5156,#2815,.T.);
#6298=EDGE_CURVE('',#5156,#5151,#4484,.T.);
#6299=EDGE_CURVE('',#5157,#5158,#2816,.T.);
#6300=EDGE_CURVE('',#5157,#5159,#2817,.T.);
#6301=EDGE_CURVE('',#5159,#5160,#2818,.T.);
#6302=EDGE_CURVE('',#5160,#5158,#2819,.T.);
#6303=EDGE_CURVE('',#5097,#5161,#2820,.T.);
#6304=EDGE_CURVE('',#5162,#5161,#2821,.T.);
#6305=EDGE_CURVE('',#5116,#5162,#2822,.T.);
#6306=EDGE_CURVE('',#5163,#5115,#2823,.T.);
#6307=EDGE_CURVE('',#5164,#5163,#2824,.T.);
#6308=EDGE_CURVE('',#5164,#5098,#2825,.T.);
#6309=EDGE_CURVE('',#5161,#5165,#4485,.T.);
#6310=EDGE_CURVE('',#5166,#5165,#2826,.T.);
#6311=EDGE_CURVE('',#5162,#5166,#4486,.T.);
#6312=EDGE_CURVE('',#5167,#5168,#2827,.T.);
#6313=EDGE_CURVE('',#5167,#5164,#751,.T.);
#6314=EDGE_CURVE('',#5168,#5163,#752,.T.);
#6315=EDGE_CURVE('',#5165,#5169,#2828,.T.);
#6316=EDGE_CURVE('',#5169,#5170,#2829,.T.);
#6317=EDGE_CURVE('',#5166,#5170,#2830,.T.);
#6318=EDGE_CURVE('',#5171,#5168,#2831,.T.);
#6319=EDGE_CURVE('',#5171,#5172,#2832,.T.);
#6320=EDGE_CURVE('',#5172,#5167,#2833,.T.);
#6321=EDGE_CURVE('',#5173,#5120,#2834,.T.);
#6322=EDGE_CURVE('',#5173,#5055,#2835,.T.);
#6323=EDGE_CURVE('',#5170,#5119,#4487,.T.);
#6324=EDGE_CURVE('',#5054,#5174,#2836,.T.);
#6325=EDGE_CURVE('',#5174,#5130,#2837,.T.);
#6326=EDGE_CURVE('',#5129,#5171,#753,.T.);
#6327=EDGE_CURVE('',#5159,#5175,#4488,.T.);
#6328=EDGE_CURVE('',#5175,#5176,#2838,.T.);
#6329=EDGE_CURVE('',#5176,#5125,#4489,.T.);
#6330=EDGE_CURVE('',#5124,#5177,#4490,.T.);
#6331=EDGE_CURVE('',#5178,#5177,#2839,.T.);
#6332=EDGE_CURVE('',#5178,#5179,#4491,.T.);
#6333=EDGE_CURVE('',#5047,#5179,#2840,.T.);
#6334=EDGE_CURVE('',#5048,#5180,#2841,.T.);
#6335=EDGE_CURVE('',#5180,#5150,#2842,.T.);
#6336=EDGE_CURVE('',#5181,#5149,#2843,.T.);
#6337=EDGE_CURVE('',#5181,#5182,#4492,.T.);
#6338=EDGE_CURVE('',#5183,#5182,#2844,.T.);
#6339=EDGE_CURVE('',#5183,#5160,#4493,.T.);
#6340=EDGE_CURVE('',#5184,#5185,#2845,.T.);
#6341=EDGE_CURVE('',#5184,#5173,#4494,.T.);
#6342=EDGE_CURVE('',#5123,#5086,#2846,.T.);
#6343=EDGE_CURVE('',#5174,#5185,#754,.T.);
#6344=EDGE_CURVE('',#5186,#5187,#2847,.T.);
#6345=EDGE_CURVE('',#5186,#5188,#4495,.T.);
#6346=EDGE_CURVE('',#5188,#5189,#2848,.T.);
#6347=EDGE_CURVE('',#5189,#5137,#4496,.T.);
#6348=EDGE_CURVE('',#5136,#5190,#4497,.T.);
#6349=EDGE_CURVE('',#5191,#5190,#2849,.T.);
#6350=EDGE_CURVE('',#5191,#5192,#4498,.T.);
#6351=EDGE_CURVE('',#5193,#5192,#2850,.T.);
#6352=EDGE_CURVE('',#5193,#5194,#4499,.T.);
#6353=EDGE_CURVE('',#5194,#5195,#2851,.T.);
#6354=EDGE_CURVE('',#5195,#5196,#4500,.T.);
#6355=EDGE_CURVE('',#5196,#5069,#4501,.T.);
#6356=EDGE_CURVE('',#5070,#5197,#4502,.T.);
#6357=EDGE_CURVE('',#5198,#5197,#2852,.T.);
#6358=EDGE_CURVE('',#5198,#5199,#4503,.T.);
#6359=EDGE_CURVE('',#5200,#5199,#2853,.T.);
#6360=EDGE_CURVE('',#5200,#5187,#4504,.T.);
#6361=EDGE_CURVE('',#5201,#5202,#2854,.T.);
#6362=EDGE_CURVE('',#5201,#5193,#2855,.T.);
#6363=EDGE_CURVE('',#5192,#5202,#2856,.T.);
#6364=EDGE_CURVE('',#5203,#5204,#2857,.T.);
#6365=EDGE_CURVE('',#5203,#5205,#2858,.T.);
#6366=EDGE_CURVE('',#5205,#5206,#2859,.T.);
#6367=EDGE_CURVE('',#5204,#5206,#2860,.T.);
#6368=EDGE_CURVE('',#5206,#5207,#4505,.T.);
#6369=EDGE_CURVE('',#5208,#5207,#2861,.T.);
#6370=EDGE_CURVE('',#5204,#5208,#4506,.T.);
#6371=EDGE_CURVE('',#5138,#5209,#4507,.T.);
#6372=EDGE_CURVE('',#5209,#5210,#2862,.T.);
#6373=EDGE_CURVE('',#5210,#5211,#4508,.T.);
#6374=EDGE_CURVE('',#5211,#5212,#2863,.T.);
#6375=EDGE_CURVE('',#5212,#5213,#4509,.T.);
#6376=EDGE_CURVE('',#5213,#5214,#2864,.T.);
#6377=EDGE_CURVE('',#5214,#5215,#4510,.T.);
#6378=EDGE_CURVE('',#5215,#5216,#2865,.T.);
#6379=EDGE_CURVE('',#5216,#5217,#4511,.T.);
#6380=EDGE_CURVE('',#5217,#5218,#2866,.T.);
#6381=EDGE_CURVE('',#5218,#5219,#2867,.T.);
#6382=EDGE_CURVE('',#5219,#5201,#4512,.T.);
#6383=EDGE_CURVE('',#5202,#5220,#4513,.T.);
#6384=EDGE_CURVE('',#5220,#5221,#2868,.T.);
#6385=EDGE_CURVE('',#5221,#5139,#4514,.T.);
#6386=EDGE_CURVE('',#5222,#5134,#2869,.T.);
#6387=EDGE_CURVE('',#5222,#5223,#4515,.T.);
#6388=EDGE_CURVE('',#5223,#5224,#2870,.T.);
#6389=EDGE_CURVE('',#5224,#5225,#755,.T.);
#6390=EDGE_CURVE('',#5225,#5140,#2871,.T.);
#6391=EDGE_CURVE('',#5135,#5144,#2872,.T.);
#6392=EDGE_CURVE('',#5190,#5221,#2873,.T.);
#6393=EDGE_CURVE('',#5220,#5191,#2874,.T.);
#6394=EDGE_CURVE('',#5211,#5186,#2875,.T.);
#6395=EDGE_CURVE('',#5187,#5212,#2876,.T.);
#6396=EDGE_CURVE('',#5213,#5200,#2877,.T.);
#6397=EDGE_CURVE('',#5199,#5214,#2878,.T.);
#6398=EDGE_CURVE('',#5215,#5198,#2879,.T.);
#6399=EDGE_CURVE('',#5197,#5216,#2880,.T.);
#6400=EDGE_CURVE('',#5226,#5227,#2881,.T.);
#6401=EDGE_CURVE('',#5226,#5222,#2882,.T.);
#6402=EDGE_CURVE('',#5133,#5203,#4516,.T.);
#6403=EDGE_CURVE('',#5208,#5227,#2883,.T.);
#6404=EDGE_CURVE('',#5228,#5229,#2884,.T.);
#6405=EDGE_CURVE('',#5228,#5226,#4517,.T.);
#6406=EDGE_CURVE('',#5227,#5229,#756,.T.);
#6407=EDGE_CURVE('',#5225,#5228,#2885,.T.);
#6408=EDGE_CURVE('',#5229,#5230,#2886,.T.);
#6409=EDGE_CURVE('',#5230,#5231,#757,.T.);
#6410=EDGE_CURVE('',#5231,#5232,#2887,.T.);
#6411=EDGE_CURVE('',#5232,#5141,#758,.T.);
#6412=EDGE_CURVE('',#5233,#5234,#4518,.T.);
#6413=EDGE_CURVE('',#5234,#5224,#2888,.T.);
#6414=EDGE_CURVE('',#5223,#5233,#2889,.T.);
#6415=EDGE_CURVE('',#5235,#5236,#2890,.T.);
#6416=EDGE_CURVE('',#5236,#5232,#2891,.T.);
#6417=EDGE_CURVE('',#5235,#5231,#2892,.T.);
#6418=EDGE_CURVE('',#5237,#5230,#2893,.T.);
#6419=EDGE_CURVE('',#5237,#5235,#759,.T.);
#6420=EDGE_CURVE('',#5207,#5238,#2894,.T.);
#6421=EDGE_CURVE('',#5238,#5239,#760,.T.);
#6422=EDGE_CURVE('',#5239,#5237,#2895,.T.);
#6423=EDGE_CURVE('',#5240,#5241,#2896,.T.);
#6424=EDGE_CURVE('',#5241,#5242,#4519,.T.);
#6425=EDGE_CURVE('',#5242,#5243,#2897,.T.);
#6426=EDGE_CURVE('',#5243,#5240,#2898,.T.);
#6427=EDGE_CURVE('',#5205,#5131,#4520,.T.);
#6428=EDGE_CURVE('',#5132,#5244,#2899,.T.);
#6429=EDGE_CURVE('',#5244,#5245,#2900,.T.);
#6430=EDGE_CURVE('',#5245,#5238,#2901,.T.);
#6431=EDGE_CURVE('',#5245,#5246,#4521,.T.);
#6432=EDGE_CURVE('',#5246,#5239,#2902,.T.);
#6433=EDGE_CURVE('',#5142,#5236,#761,.T.);
#6434=EDGE_CURVE('',#5246,#5247,#2903,.T.);
#6435=EDGE_CURVE('',#5247,#5143,#2904,.T.);
#6436=EDGE_CURVE('',#5248,#5249,#2905,.T.);
#6437=EDGE_CURVE('',#5249,#5250,#2906,.T.);
#6438=EDGE_CURVE('',#5250,#5251,#2907,.T.);
#6439=EDGE_CURVE('',#5251,#5248,#2908,.T.);
#6440=EDGE_CURVE('',#5196,#5252,#2909,.T.);
#6441=EDGE_CURVE('',#5252,#5253,#762,.T.);
#6442=EDGE_CURVE('',#5253,#5217,#854,.T.);
#6443=EDGE_CURVE('',#5069,#5070,#4522,.T.);
#6444=EDGE_CURVE('',#5254,#5255,#2910,.T.);
#6445=EDGE_CURVE('',#5254,#5256,#2911,.T.);
#6446=EDGE_CURVE('',#5256,#5257,#2912,.T.);
#6447=EDGE_CURVE('',#5257,#5255,#2913,.T.);
#6448=EDGE_CURVE('',#5258,#5259,#2914,.T.);
#6449=EDGE_CURVE('',#5258,#5260,#2915,.T.);
#6450=EDGE_CURVE('',#5261,#5260,#2916,.T.);
#6451=EDGE_CURVE('',#5261,#5257,#4523,.T.);
#6452=EDGE_CURVE('',#5256,#5259,#4524,.T.);
#6453=EDGE_CURVE('',#5219,#5262,#2917,.T.);
#6454=EDGE_CURVE('',#5218,#5258,#763,.T.);
#6455=EDGE_CURVE('',#5259,#5262,#2918,.T.);
#6456=EDGE_CURVE('',#5263,#5264,#2919,.T.);
#6457=EDGE_CURVE('',#5264,#5265,#2920,.T.);
#6458=EDGE_CURVE('',#5265,#5266,#4525,.T.);
#6459=EDGE_CURVE('',#5263,#5266,#2921,.T.);
#6460=EDGE_CURVE('',#5267,#5263,#2922,.T.);
#6461=EDGE_CURVE('',#5267,#5261,#2923,.T.);
#6462=EDGE_CURVE('',#5260,#5253,#764,.T.);
#6463=EDGE_CURVE('',#5252,#5264,#765,.T.);
#6464=EDGE_CURVE('',#5266,#5268,#2924,.T.);
#6465=EDGE_CURVE('',#5268,#5219,#2925,.T.);
#6466=EDGE_CURVE('',#5262,#5254,#4526,.T.);
#6467=EDGE_CURVE('',#5255,#5267,#4527,.T.);
#6468=EDGE_CURVE('',#5177,#5269,#2926,.T.);
#6469=EDGE_CURVE('',#5270,#5269,#2927,.T.);
#6470=EDGE_CURVE('',#5270,#5178,#2928,.T.);
#6471=EDGE_CURVE('',#5049,#5271,#2929,.T.);
#6472=EDGE_CURVE('',#5179,#5271,#2930,.T.);
#6473=EDGE_CURVE('',#5272,#5148,#2931,.T.);
#6474=EDGE_CURVE('',#5272,#5181,#2932,.T.);
#6475=EDGE_CURVE('',#5273,#5274,#2933,.T.);
#6476=EDGE_CURVE('',#5273,#5183,#2934,.T.);
#6477=EDGE_CURVE('',#5182,#5274,#2935,.T.);
#6478=EDGE_CURVE('',#5126,#5275,#4528,.T.);
#6479=EDGE_CURVE('',#5275,#5276,#2936,.T.);
#6480=EDGE_CURVE('',#5276,#5157,#4529,.T.);
#6481=EDGE_CURVE('',#5158,#5273,#4530,.T.);
#6482=EDGE_CURVE('',#5274,#5272,#4531,.T.);
#6483=EDGE_CURVE('',#5147,#5277,#4532,.T.);
#6484=EDGE_CURVE('',#5277,#5050,#2937,.T.);
#6485=EDGE_CURVE('',#5271,#5270,#4533,.T.);
#6486=EDGE_CURVE('',#5269,#5127,#4534,.T.);
#6487=EDGE_CURVE('',#5185,#5052,#2938,.T.);
#6488=EDGE_CURVE('',#5053,#5184,#2939,.T.);
#6489=EDGE_CURVE('',#5087,#5278,#2940,.T.);
#6490=EDGE_CURVE('',#5279,#5085,#2941,.T.);
#6491=EDGE_CURVE('',#5279,#5280,#2942,.T.);
#6492=EDGE_CURVE('',#5280,#5278,#766,.T.);
#6493=EDGE_CURVE('',#5121,#5169,#4535,.T.);
#6494=EDGE_CURVE('',#5093,#5281,#2943,.T.);
#6495=EDGE_CURVE('',#5281,#5122,#2944,.T.);
#6496=EDGE_CURVE('',#5172,#5128,#767,.T.);
#6497=EDGE_CURVE('',#5089,#5094,#2945,.T.);
#6498=EDGE_CURVE('',#5092,#5088,#2946,.T.);
#6499=EDGE_CURVE('',#5278,#5091,#2947,.T.);
#6500=EDGE_CURVE('',#5282,#5283,#4536,.T.);
#6501=EDGE_CURVE('',#5283,#5284,#2948,.T.);
#6502=EDGE_CURVE('',#5285,#5284,#2949,.T.);
#6503=EDGE_CURVE('',#5285,#5282,#2950,.T.);
#6504=EDGE_CURVE('',#5151,#5286,#2951,.T.);
#6505=EDGE_CURVE('',#5286,#5285,#2952,.T.);
#6506=EDGE_CURVE('',#5284,#5145,#768,.T.);
#6507=EDGE_CURVE('',#5146,#5152,#769,.T.);
#6508=EDGE_CURVE('',#5155,#5287,#2953,.T.);
#6509=EDGE_CURVE('',#5287,#5288,#2954,.T.);
#6510=EDGE_CURVE('',#5288,#5156,#2955,.T.);
#6511=EDGE_CURVE('',#5048,#5289,#2956,.T.);
#6512=EDGE_CURVE('',#5289,#5154,#2957,.T.);
#6513=EDGE_CURVE('',#5153,#5180,#770,.T.);
#6514=EDGE_CURVE('',#5051,#5282,#2958,.T.);
#6515=EDGE_CURVE('',#5286,#5288,#4537,.T.);
#6516=EDGE_CURVE('',#5287,#5289,#4538,.T.);
#6517=EDGE_CURVE('',#5144,#5249,#4539,.T.);
#6518=EDGE_CURVE('',#5248,#5135,#4540,.T.);
#6519=EDGE_CURVE('',#5290,#5291,#2959,.T.);
#6520=EDGE_CURVE('',#5290,#5292,#2960,.T.);
#6521=EDGE_CURVE('',#5292,#5293,#2961,.T.);
#6522=EDGE_CURVE('',#5293,#5291,#2962,.T.);
#6523=EDGE_CURVE('',#5123,#5279,#4541,.T.);
#6524=EDGE_CURVE('',#5294,#5295,#2963,.T.);
#6525=EDGE_CURVE('',#5294,#5296,#2964,.T.);
#6526=EDGE_CURVE('',#5296,#5297,#2965,.T.);
#6527=EDGE_CURVE('',#5297,#5295,#2966,.T.);
#6528=EDGE_CURVE('',#5296,#5298,#4542,.T.);
#6529=EDGE_CURVE('',#5298,#5299,#2967,.T.);
#6530=EDGE_CURVE('',#5299,#5293,#4543,.T.);
#6531=EDGE_CURVE('',#5292,#5300,#4544,.T.);
#6532=EDGE_CURVE('',#5300,#5301,#2968,.T.);
#6533=EDGE_CURVE('',#5301,#5297,#4545,.T.);
#6534=EDGE_CURVE('',#5302,#5303,#2969,.T.);
#6535=EDGE_CURVE('',#5303,#5294,#4546,.T.);
#6536=EDGE_CURVE('',#5295,#5304,#4547,.T.);
#6537=EDGE_CURVE('',#5304,#5305,#2970,.T.);
#6538=EDGE_CURVE('',#5305,#5290,#4548,.T.);
#6539=EDGE_CURVE('',#5291,#5302,#4549,.T.);
#6540=EDGE_CURVE('',#5280,#5281,#771,.T.);
#6541=EDGE_CURVE('',#5244,#5251,#4550,.T.);
#6542=EDGE_CURVE('',#5250,#5247,#4551,.T.);
#6543=EDGE_CURVE('',#5251,#5243,#4552,.T.);
#6544=EDGE_CURVE('',#5240,#5250,#4553,.T.);
#6545=EDGE_CURVE('',#5244,#5243,#4554,.T.);
#6546=EDGE_CURVE('',#5240,#5247,#4555,.T.);
#6547=EDGE_CURVE('',#5245,#5242,#4556,.T.);
#6548=EDGE_CURVE('',#5241,#5246,#4557,.T.);
#6549=EDGE_CURVE('',#5277,#5283,#855,.T.);
#6550=EDGE_CURVE('',#5265,#5195,#856,.T.);
#6551=EDGE_CURVE('',#5194,#5268,#857,.T.);
#6552=EDGE_CURVE('',#5305,#5276,#858,.T.);
#6553=EDGE_CURVE('',#5275,#5300,#859,.T.);
#6554=EDGE_CURVE('',#5299,#5189,#860,.T.);
#6555=EDGE_CURVE('',#5188,#5302,#861,.T.);
#6556=EDGE_CURVE('',#5233,#5226,#4558,.T.);
#6557=EDGE_CURVE('',#5234,#5228,#4559,.T.);
#6558=EDGE_CURVE('',#5298,#5209,#862,.T.);
#6559=EDGE_CURVE('',#5176,#5301,#863,.T.);
#6560=EDGE_CURVE('',#5304,#5175,#864,.T.);
#6561=EDGE_CURVE('',#5210,#5303,#865,.T.);
#7851=ORIENTED_EDGE('',*,*,#6138,.F.);
#7852=ORIENTED_EDGE('',*,*,#6139,.T.);
#7853=ORIENTED_EDGE('',*,*,#6140,.F.);
#7854=ORIENTED_EDGE('',*,*,#6139,.F.);
#7855=ORIENTED_EDGE('',*,*,#6141,.F.);
#7856=ORIENTED_EDGE('',*,*,#6142,.T.);
#7857=ORIENTED_EDGE('',*,*,#6143,.F.);
#7858=ORIENTED_EDGE('',*,*,#6142,.F.);
#7859=ORIENTED_EDGE('',*,*,#6144,.F.);
#7860=ORIENTED_EDGE('',*,*,#6145,.T.);
#7861=ORIENTED_EDGE('',*,*,#6146,.F.);
#7862=ORIENTED_EDGE('',*,*,#6145,.F.);
#7863=ORIENTED_EDGE('',*,*,#6147,.F.);
#7864=ORIENTED_EDGE('',*,*,#6148,.T.);
#7865=ORIENTED_EDGE('',*,*,#6149,.F.);
#7866=ORIENTED_EDGE('',*,*,#6148,.F.);
#7867=ORIENTED_EDGE('',*,*,#6150,.F.);
#7868=ORIENTED_EDGE('',*,*,#6151,.T.);
#7869=ORIENTED_EDGE('',*,*,#6152,.F.);
#7870=ORIENTED_EDGE('',*,*,#6151,.F.);
#7871=ORIENTED_EDGE('',*,*,#6153,.F.);
#7872=ORIENTED_EDGE('',*,*,#6154,.T.);
#7873=ORIENTED_EDGE('',*,*,#6155,.F.);
#7874=ORIENTED_EDGE('',*,*,#6154,.F.);
#7875=ORIENTED_EDGE('',*,*,#6156,.F.);
#7876=ORIENTED_EDGE('',*,*,#6157,.F.);
#7877=ORIENTED_EDGE('',*,*,#6158,.F.);
#7878=ORIENTED_EDGE('',*,*,#6159,.F.);
#7879=ORIENTED_EDGE('',*,*,#6160,.T.);
#7880=ORIENTED_EDGE('',*,*,#6161,.F.);
#7881=ORIENTED_EDGE('',*,*,#6162,.F.);
#7882=ORIENTED_EDGE('',*,*,#6163,.F.);
#7883=ORIENTED_EDGE('',*,*,#6164,.T.);
#7884=ORIENTED_EDGE('',*,*,#6165,.F.);
#7885=ORIENTED_EDGE('',*,*,#6166,.T.);
#7886=ORIENTED_EDGE('',*,*,#6167,.F.);
#7887=ORIENTED_EDGE('',*,*,#6166,.F.);
#7888=ORIENTED_EDGE('',*,*,#6168,.F.);
#7889=ORIENTED_EDGE('',*,*,#6169,.T.);
#7890=ORIENTED_EDGE('',*,*,#6170,.F.);
#7891=ORIENTED_EDGE('',*,*,#6169,.F.);
#7892=ORIENTED_EDGE('',*,*,#6171,.F.);
#7893=ORIENTED_EDGE('',*,*,#6172,.T.);
#7894=ORIENTED_EDGE('',*,*,#6173,.F.);
#7895=ORIENTED_EDGE('',*,*,#6172,.F.);
#7896=ORIENTED_EDGE('',*,*,#6174,.F.);
#7897=ORIENTED_EDGE('',*,*,#6175,.T.);
#7898=ORIENTED_EDGE('',*,*,#6176,.F.);
#7899=ORIENTED_EDGE('',*,*,#6175,.F.);
#7900=ORIENTED_EDGE('',*,*,#6177,.F.);
#7901=ORIENTED_EDGE('',*,*,#6178,.F.);
#7902=ORIENTED_EDGE('',*,*,#6179,.F.);
#7903=ORIENTED_EDGE('',*,*,#6180,.F.);
#7904=ORIENTED_EDGE('',*,*,#6181,.F.);
#7905=ORIENTED_EDGE('',*,*,#6182,.F.);
#7906=ORIENTED_EDGE('',*,*,#6183,.F.);
#7907=ORIENTED_EDGE('',*,*,#6184,.F.);
#7908=ORIENTED_EDGE('',*,*,#6185,.F.);
#7909=ORIENTED_EDGE('',*,*,#6186,.F.);
#7910=ORIENTED_EDGE('',*,*,#6187,.F.);
#7911=ORIENTED_EDGE('',*,*,#6188,.T.);
#7912=ORIENTED_EDGE('',*,*,#6189,.F.);
#7913=ORIENTED_EDGE('',*,*,#6190,.F.);
#7914=ORIENTED_EDGE('',*,*,#6188,.F.);
#7915=ORIENTED_EDGE('',*,*,#6191,.F.);
#7916=ORIENTED_EDGE('',*,*,#6192,.T.);
#7917=ORIENTED_EDGE('',*,*,#6193,.F.);
#7918=ORIENTED_EDGE('',*,*,#6192,.F.);
#7919=ORIENTED_EDGE('',*,*,#6194,.F.);
#7920=ORIENTED_EDGE('',*,*,#6195,.F.);
#7921=ORIENTED_EDGE('',*,*,#6196,.T.);
#7922=ORIENTED_EDGE('',*,*,#6197,.F.);
#7923=ORIENTED_EDGE('',*,*,#6196,.F.);
#7924=ORIENTED_EDGE('',*,*,#6198,.F.);
#7925=ORIENTED_EDGE('',*,*,#6199,.F.);
#7926=ORIENTED_EDGE('',*,*,#6200,.T.);
#7927=ORIENTED_EDGE('',*,*,#6201,.F.);
#7928=ORIENTED_EDGE('',*,*,#6200,.F.);
#7929=ORIENTED_EDGE('',*,*,#6202,.F.);
#7930=ORIENTED_EDGE('',*,*,#6203,.F.);
#7931=ORIENTED_EDGE('',*,*,#6204,.F.);
#7932=ORIENTED_EDGE('',*,*,#6205,.T.);
#7933=ORIENTED_EDGE('',*,*,#6206,.F.);
#7934=ORIENTED_EDGE('',*,*,#6207,.F.);
#7935=ORIENTED_EDGE('',*,*,#6208,.F.);
#7936=ORIENTED_EDGE('',*,*,#6209,.T.);
#7937=ORIENTED_EDGE('',*,*,#6210,.F.);
#7938=ORIENTED_EDGE('',*,*,#6211,.F.);
#7939=ORIENTED_EDGE('',*,*,#6212,.T.);
#7940=ORIENTED_EDGE('',*,*,#6213,.T.);
#7941=ORIENTED_EDGE('',*,*,#6214,.T.);
#7942=ORIENTED_EDGE('',*,*,#6213,.F.);
#7943=ORIENTED_EDGE('',*,*,#6173,.T.);
#7944=ORIENTED_EDGE('',*,*,#6215,.T.);
#7945=ORIENTED_EDGE('',*,*,#6144,.T.);
#7946=ORIENTED_EDGE('',*,*,#6215,.F.);
#7947=ORIENTED_EDGE('',*,*,#6180,.T.);
#7948=ORIENTED_EDGE('',*,*,#6216,.T.);
#7949=ORIENTED_EDGE('',*,*,#6138,.T.);
#7950=ORIENTED_EDGE('',*,*,#6216,.F.);
#7951=ORIENTED_EDGE('',*,*,#6179,.T.);
#7952=ORIENTED_EDGE('',*,*,#6217,.T.);
#7953=ORIENTED_EDGE('',*,*,#6176,.T.);
#7954=ORIENTED_EDGE('',*,*,#6218,.T.);
#7955=ORIENTED_EDGE('',*,*,#6147,.T.);
#7956=ORIENTED_EDGE('',*,*,#6218,.F.);
#7957=ORIENTED_EDGE('',*,*,#6210,.T.);
#7958=ORIENTED_EDGE('',*,*,#6219,.T.);
#7959=ORIENTED_EDGE('',*,*,#6220,.F.);
#7960=ORIENTED_EDGE('',*,*,#6221,.F.);
#7961=ORIENTED_EDGE('',*,*,#6198,.T.);
#7962=ORIENTED_EDGE('',*,*,#6199,.T.);
#7963=ORIENTED_EDGE('',*,*,#6222,.T.);
#7964=ORIENTED_EDGE('',*,*,#6223,.T.);
#7965=ORIENTED_EDGE('',*,*,#6222,.F.);
#7966=ORIENTED_EDGE('',*,*,#6224,.F.);
#7967=ORIENTED_EDGE('',*,*,#6225,.T.);
#7968=ORIENTED_EDGE('',*,*,#6226,.F.);
#7969=ORIENTED_EDGE('',*,*,#6225,.F.);
#7970=ORIENTED_EDGE('',*,*,#6227,.F.);
#7971=ORIENTED_EDGE('',*,*,#6228,.T.);
#7972=ORIENTED_EDGE('',*,*,#6229,.F.);
#7973=ORIENTED_EDGE('',*,*,#6228,.F.);
#7974=ORIENTED_EDGE('',*,*,#6230,.F.);
#7975=ORIENTED_EDGE('',*,*,#6231,.T.);
#7976=ORIENTED_EDGE('',*,*,#6232,.F.);
#7977=ORIENTED_EDGE('',*,*,#6231,.F.);
#7978=ORIENTED_EDGE('',*,*,#6170,.T.);
#7979=ORIENTED_EDGE('',*,*,#6233,.T.);
#7980=ORIENTED_EDGE('',*,*,#6150,.T.);
#7981=ORIENTED_EDGE('',*,*,#6233,.F.);
#7982=ORIENTED_EDGE('',*,*,#6185,.T.);
#7983=ORIENTED_EDGE('',*,*,#6234,.T.);
#7984=ORIENTED_EDGE('',*,*,#6141,.T.);
#7985=ORIENTED_EDGE('',*,*,#6234,.F.);
#7986=ORIENTED_EDGE('',*,*,#6184,.T.);
#7987=ORIENTED_EDGE('',*,*,#6235,.T.);
#7988=ORIENTED_EDGE('',*,*,#6167,.T.);
#7989=ORIENTED_EDGE('',*,*,#6236,.T.);
#7990=ORIENTED_EDGE('',*,*,#6153,.T.);
#7991=ORIENTED_EDGE('',*,*,#6236,.F.);
#7992=ORIENTED_EDGE('',*,*,#6194,.T.);
#7993=ORIENTED_EDGE('',*,*,#6195,.T.);
#7994=ORIENTED_EDGE('',*,*,#6237,.T.);
#7995=ORIENTED_EDGE('',*,*,#6238,.F.);
#7996=ORIENTED_EDGE('',*,*,#6237,.F.);
#7997=ORIENTED_EDGE('',*,*,#6239,.T.);
#7998=ORIENTED_EDGE('',*,*,#6240,.T.);
#7999=ORIENTED_EDGE('',*,*,#6241,.T.);
#8000=ORIENTED_EDGE('',*,*,#6240,.F.);
#8001=ORIENTED_EDGE('',*,*,#6242,.T.);
#8002=ORIENTED_EDGE('',*,*,#6243,.T.);
#8003=ORIENTED_EDGE('',*,*,#6244,.T.);
#8004=ORIENTED_EDGE('',*,*,#6243,.F.);
#8005=ORIENTED_EDGE('',*,*,#6245,.T.);
#8006=ORIENTED_EDGE('',*,*,#6246,.T.);
#8007=ORIENTED_EDGE('',*,*,#6247,.T.);
#8008=ORIENTED_EDGE('',*,*,#6246,.F.);
#8009=ORIENTED_EDGE('',*,*,#6193,.T.);
#8010=ORIENTED_EDGE('',*,*,#6248,.T.);
#8011=ORIENTED_EDGE('',*,*,#6189,.T.);
#8012=ORIENTED_EDGE('',*,*,#6190,.T.);
#8013=ORIENTED_EDGE('',*,*,#6248,.F.);
#8014=ORIENTED_EDGE('',*,*,#6249,.F.);
#8015=ORIENTED_EDGE('',*,*,#6250,.T.);
#8016=ORIENTED_EDGE('',*,*,#6251,.F.);
#8017=ORIENTED_EDGE('',*,*,#6250,.F.);
#8018=ORIENTED_EDGE('',*,*,#6163,.T.);
#8019=ORIENTED_EDGE('',*,*,#6252,.T.);
#8020=ORIENTED_EDGE('',*,*,#6253,.T.);
#8021=ORIENTED_EDGE('',*,*,#6254,.F.);
#8022=ORIENTED_EDGE('',*,*,#6255,.T.);
#8023=ORIENTED_EDGE('',*,*,#6256,.T.);
#8024=ORIENTED_EDGE('',*,*,#6257,.T.);
#8025=ORIENTED_EDGE('',*,*,#6256,.F.);
#8026=ORIENTED_EDGE('',*,*,#6258,.F.);
#8027=ORIENTED_EDGE('',*,*,#6259,.T.);
#8028=ORIENTED_EDGE('',*,*,#6260,.T.);
#8029=ORIENTED_EDGE('',*,*,#6261,.T.);
#8030=ORIENTED_EDGE('',*,*,#6262,.F.);
#8031=ORIENTED_EDGE('',*,*,#6263,.T.);
#8032=ORIENTED_EDGE('',*,*,#6264,.T.);
#8033=ORIENTED_EDGE('',*,*,#6265,.F.);
#8034=ORIENTED_EDGE('',*,*,#6266,.T.);
#8035=ORIENTED_EDGE('',*,*,#6267,.T.);
#8036=ORIENTED_EDGE('',*,*,#6268,.T.);
#8037=ORIENTED_EDGE('',*,*,#6269,.F.);
#8038=ORIENTED_EDGE('',*,*,#6270,.F.);
#8039=ORIENTED_EDGE('',*,*,#6207,.T.);
#8040=ORIENTED_EDGE('',*,*,#6271,.F.);
#8041=ORIENTED_EDGE('',*,*,#6272,.T.);
#8042=ORIENTED_EDGE('',*,*,#6273,.T.);
#8043=ORIENTED_EDGE('',*,*,#6274,.T.);
#8044=ORIENTED_EDGE('',*,*,#6275,.T.);
#8045=ORIENTED_EDGE('',*,*,#6276,.T.);
#8046=ORIENTED_EDGE('',*,*,#6277,.T.);
#8047=ORIENTED_EDGE('',*,*,#6278,.F.);
#8048=ORIENTED_EDGE('',*,*,#6279,.T.);
#8049=ORIENTED_EDGE('',*,*,#6280,.T.);
#8050=ORIENTED_EDGE('',*,*,#6281,.T.);
#8051=ORIENTED_EDGE('',*,*,#6282,.F.);
#8052=ORIENTED_EDGE('',*,*,#6283,.T.);
#8053=ORIENTED_EDGE('',*,*,#6284,.T.);
#8054=ORIENTED_EDGE('',*,*,#6285,.F.);
#8055=ORIENTED_EDGE('',*,*,#6286,.T.);
#8056=ORIENTED_EDGE('',*,*,#6287,.F.);
#8057=ORIENTED_EDGE('',*,*,#6288,.F.);
#8058=ORIENTED_EDGE('',*,*,#6289,.F.);
#8059=ORIENTED_EDGE('',*,*,#6290,.F.);
#8060=ORIENTED_EDGE('',*,*,#6291,.F.);
#8061=ORIENTED_EDGE('',*,*,#6292,.T.);
#8062=ORIENTED_EDGE('',*,*,#6293,.T.);
#8063=ORIENTED_EDGE('',*,*,#6294,.T.);
#8064=ORIENTED_EDGE('',*,*,#6295,.T.);
#8065=ORIENTED_EDGE('',*,*,#6296,.T.);
#8066=ORIENTED_EDGE('',*,*,#6297,.T.);
#8067=ORIENTED_EDGE('',*,*,#6298,.T.);
#8068=ORIENTED_EDGE('',*,*,#6299,.F.);
#8069=ORIENTED_EDGE('',*,*,#6300,.T.);
#8070=ORIENTED_EDGE('',*,*,#6301,.T.);
#8071=ORIENTED_EDGE('',*,*,#6302,.T.);
#8072=ORIENTED_EDGE('',*,*,#6220,.T.);
#8073=ORIENTED_EDGE('',*,*,#6303,.T.);
#8074=ORIENTED_EDGE('',*,*,#6304,.F.);
#8075=ORIENTED_EDGE('',*,*,#6305,.F.);
#8076=ORIENTED_EDGE('',*,*,#6253,.F.);
#8077=ORIENTED_EDGE('',*,*,#6306,.F.);
#8078=ORIENTED_EDGE('',*,*,#6307,.F.);
#8079=ORIENTED_EDGE('',*,*,#6308,.T.);
#8080=ORIENTED_EDGE('',*,*,#6304,.T.);
#8081=ORIENTED_EDGE('',*,*,#6309,.T.);
#8082=ORIENTED_EDGE('',*,*,#6310,.F.);
#8083=ORIENTED_EDGE('',*,*,#6311,.F.);
#8084=ORIENTED_EDGE('',*,*,#6312,.F.);
#8085=ORIENTED_EDGE('',*,*,#6313,.T.);
#8086=ORIENTED_EDGE('',*,*,#6307,.T.);
#8087=ORIENTED_EDGE('',*,*,#6314,.F.);
#8088=ORIENTED_EDGE('',*,*,#6315,.T.);
#8089=ORIENTED_EDGE('',*,*,#6316,.T.);
#8090=ORIENTED_EDGE('',*,*,#6317,.F.);
#8091=ORIENTED_EDGE('',*,*,#6310,.T.);
#8092=ORIENTED_EDGE('',*,*,#6318,.F.);
#8093=ORIENTED_EDGE('',*,*,#6319,.T.);
#8094=ORIENTED_EDGE('',*,*,#6320,.T.);
#8095=ORIENTED_EDGE('',*,*,#6312,.T.);
#8096=ORIENTED_EDGE('',*,*,#6321,.F.);
#8097=ORIENTED_EDGE('',*,*,#6322,.T.);
#8098=ORIENTED_EDGE('',*,*,#6254,.T.);
#8099=ORIENTED_EDGE('',*,*,#6305,.T.);
#8100=ORIENTED_EDGE('',*,*,#6311,.T.);
#8101=ORIENTED_EDGE('',*,*,#6317,.T.);
#8102=ORIENTED_EDGE('',*,*,#6323,.T.);
#8103=ORIENTED_EDGE('',*,*,#6258,.T.);
#8104=ORIENTED_EDGE('',*,*,#6252,.F.);
#8105=ORIENTED_EDGE('',*,*,#6324,.T.);
#8106=ORIENTED_EDGE('',*,*,#6325,.T.);
#8107=ORIENTED_EDGE('',*,*,#6269,.T.);
#8108=ORIENTED_EDGE('',*,*,#6326,.T.);
#8109=ORIENTED_EDGE('',*,*,#6318,.T.);
#8110=ORIENTED_EDGE('',*,*,#6314,.T.);
#8111=ORIENTED_EDGE('',*,*,#6306,.T.);
#8112=ORIENTED_EDGE('',*,*,#6327,.T.);
#8113=ORIENTED_EDGE('',*,*,#6328,.T.);
#8114=ORIENTED_EDGE('',*,*,#6329,.T.);
#8115=ORIENTED_EDGE('',*,*,#6263,.F.);
#8116=ORIENTED_EDGE('',*,*,#6330,.T.);
#8117=ORIENTED_EDGE('',*,*,#6331,.F.);
#8118=ORIENTED_EDGE('',*,*,#6332,.T.);
#8119=ORIENTED_EDGE('',*,*,#6333,.F.);
#8120=ORIENTED_EDGE('',*,*,#6156,.T.);
#8121=ORIENTED_EDGE('',*,*,#6334,.T.);
#8122=ORIENTED_EDGE('',*,*,#6335,.T.);
#8123=ORIENTED_EDGE('',*,*,#6291,.T.);
#8124=ORIENTED_EDGE('',*,*,#6336,.F.);
#8125=ORIENTED_EDGE('',*,*,#6337,.T.);
#8126=ORIENTED_EDGE('',*,*,#6338,.F.);
#8127=ORIENTED_EDGE('',*,*,#6339,.T.);
#8128=ORIENTED_EDGE('',*,*,#6301,.F.);
#8129=ORIENTED_EDGE('',*,*,#6224,.T.);
#8130=ORIENTED_EDGE('',*,*,#6227,.T.);
#8131=ORIENTED_EDGE('',*,*,#6230,.T.);
#8132=ORIENTED_EDGE('',*,*,#6201,.T.);
#8133=ORIENTED_EDGE('',*,*,#6340,.F.);
#8134=ORIENTED_EDGE('',*,*,#6341,.T.);
#8135=ORIENTED_EDGE('',*,*,#6321,.T.);
#8136=ORIENTED_EDGE('',*,*,#6262,.T.);
#8137=ORIENTED_EDGE('',*,*,#6342,.T.);
#8138=ORIENTED_EDGE('',*,*,#6270,.T.);
#8139=ORIENTED_EDGE('',*,*,#6325,.F.);
#8140=ORIENTED_EDGE('',*,*,#6343,.T.);
#8141=ORIENTED_EDGE('',*,*,#6344,.F.);
#8142=ORIENTED_EDGE('',*,*,#6345,.T.);
#8143=ORIENTED_EDGE('',*,*,#6346,.T.);
#8144=ORIENTED_EDGE('',*,*,#6347,.T.);
#8145=ORIENTED_EDGE('',*,*,#6276,.F.);
#8146=ORIENTED_EDGE('',*,*,#6348,.T.);
#8147=ORIENTED_EDGE('',*,*,#6349,.F.);
#8148=ORIENTED_EDGE('',*,*,#6350,.T.);
#8149=ORIENTED_EDGE('',*,*,#6351,.F.);
#8150=ORIENTED_EDGE('',*,*,#6352,.T.);
#8151=ORIENTED_EDGE('',*,*,#6353,.T.);
#8152=ORIENTED_EDGE('',*,*,#6354,.T.);
#8153=ORIENTED_EDGE('',*,*,#6355,.T.);
#8154=ORIENTED_EDGE('',*,*,#6182,.T.);
#8155=ORIENTED_EDGE('',*,*,#6356,.T.);
#8156=ORIENTED_EDGE('',*,*,#6357,.F.);
#8157=ORIENTED_EDGE('',*,*,#6358,.T.);
#8158=ORIENTED_EDGE('',*,*,#6359,.F.);
#8159=ORIENTED_EDGE('',*,*,#6360,.T.);
#8160=ORIENTED_EDGE('',*,*,#6168,.T.);
#8161=ORIENTED_EDGE('',*,*,#6165,.T.);
#8162=ORIENTED_EDGE('',*,*,#6187,.T.);
#8163=ORIENTED_EDGE('',*,*,#6361,.F.);
#8164=ORIENTED_EDGE('',*,*,#6362,.T.);
#8165=ORIENTED_EDGE('',*,*,#6351,.T.);
#8166=ORIENTED_EDGE('',*,*,#6363,.T.);
#8167=ORIENTED_EDGE('',*,*,#6364,.F.);
#8168=ORIENTED_EDGE('',*,*,#6365,.T.);
#8169=ORIENTED_EDGE('',*,*,#6366,.T.);
#8170=ORIENTED_EDGE('',*,*,#6367,.F.);
#8171=ORIENTED_EDGE('',*,*,#6367,.T.);
#8172=ORIENTED_EDGE('',*,*,#6368,.T.);
#8173=ORIENTED_EDGE('',*,*,#6369,.F.);
#8174=ORIENTED_EDGE('',*,*,#6370,.F.);
#8175=ORIENTED_EDGE('',*,*,#6371,.T.);
#8176=ORIENTED_EDGE('',*,*,#6372,.T.);
#8177=ORIENTED_EDGE('',*,*,#6373,.T.);
#8178=ORIENTED_EDGE('',*,*,#6374,.T.);
#8179=ORIENTED_EDGE('',*,*,#6375,.T.);
#8180=ORIENTED_EDGE('',*,*,#6376,.T.);
#8181=ORIENTED_EDGE('',*,*,#6377,.T.);
#8182=ORIENTED_EDGE('',*,*,#6378,.T.);
#8183=ORIENTED_EDGE('',*,*,#6379,.T.);
#8184=ORIENTED_EDGE('',*,*,#6380,.T.);
#8185=ORIENTED_EDGE('',*,*,#6381,.T.);
#8186=ORIENTED_EDGE('',*,*,#6382,.T.);
#8187=ORIENTED_EDGE('',*,*,#6361,.T.);
#8188=ORIENTED_EDGE('',*,*,#6383,.T.);
#8189=ORIENTED_EDGE('',*,*,#6384,.T.);
#8190=ORIENTED_EDGE('',*,*,#6385,.T.);
#8191=ORIENTED_EDGE('',*,*,#6278,.T.);
#8192=ORIENTED_EDGE('',*,*,#6242,.F.);
#8193=ORIENTED_EDGE('',*,*,#6245,.F.);
#8194=ORIENTED_EDGE('',*,*,#6239,.F.);
#8195=ORIENTED_EDGE('',*,*,#6197,.T.);
#8196=ORIENTED_EDGE('',*,*,#6274,.F.);
#8197=ORIENTED_EDGE('',*,*,#6386,.F.);
#8198=ORIENTED_EDGE('',*,*,#6387,.T.);
#8199=ORIENTED_EDGE('',*,*,#6388,.T.);
#8200=ORIENTED_EDGE('',*,*,#6389,.T.);
#8201=ORIENTED_EDGE('',*,*,#6390,.T.);
#8202=ORIENTED_EDGE('',*,*,#6284,.F.);
#8203=ORIENTED_EDGE('',*,*,#6391,.F.);
#8204=ORIENTED_EDGE('',*,*,#6349,.T.);
#8205=ORIENTED_EDGE('',*,*,#6392,.T.);
#8206=ORIENTED_EDGE('',*,*,#6384,.F.);
#8207=ORIENTED_EDGE('',*,*,#6393,.T.);
#8208=ORIENTED_EDGE('',*,*,#6374,.F.);
#8209=ORIENTED_EDGE('',*,*,#6394,.T.);
#8210=ORIENTED_EDGE('',*,*,#6344,.T.);
#8211=ORIENTED_EDGE('',*,*,#6395,.T.);
#8212=ORIENTED_EDGE('',*,*,#6376,.F.);
#8213=ORIENTED_EDGE('',*,*,#6396,.T.);
#8214=ORIENTED_EDGE('',*,*,#6359,.T.);
#8215=ORIENTED_EDGE('',*,*,#6397,.T.);
#8216=ORIENTED_EDGE('',*,*,#6378,.F.);
#8217=ORIENTED_EDGE('',*,*,#6398,.T.);
#8218=ORIENTED_EDGE('',*,*,#6357,.T.);
#8219=ORIENTED_EDGE('',*,*,#6399,.T.);
#8220=ORIENTED_EDGE('',*,*,#6238,.T.);
#8221=ORIENTED_EDGE('',*,*,#6214,.F.);
#8222=ORIENTED_EDGE('',*,*,#6400,.F.);
#8223=ORIENTED_EDGE('',*,*,#6401,.T.);
#8224=ORIENTED_EDGE('',*,*,#6386,.T.);
#8225=ORIENTED_EDGE('',*,*,#6273,.F.);
#8226=ORIENTED_EDGE('',*,*,#6402,.T.);
#8227=ORIENTED_EDGE('',*,*,#6364,.T.);
#8228=ORIENTED_EDGE('',*,*,#6370,.T.);
#8229=ORIENTED_EDGE('',*,*,#6403,.T.);
#8230=ORIENTED_EDGE('',*,*,#6404,.F.);
#8231=ORIENTED_EDGE('',*,*,#6405,.T.);
#8232=ORIENTED_EDGE('',*,*,#6400,.T.);
#8233=ORIENTED_EDGE('',*,*,#6406,.T.);
#8234=ORIENTED_EDGE('',*,*,#6390,.F.);
#8235=ORIENTED_EDGE('',*,*,#6407,.T.);
#8236=ORIENTED_EDGE('',*,*,#6404,.T.);
#8237=ORIENTED_EDGE('',*,*,#6408,.T.);
#8238=ORIENTED_EDGE('',*,*,#6409,.T.);
#8239=ORIENTED_EDGE('',*,*,#6410,.T.);
#8240=ORIENTED_EDGE('',*,*,#6411,.T.);
#8241=ORIENTED_EDGE('',*,*,#6280,.F.);
#8242=ORIENTED_EDGE('',*,*,#6412,.T.);
#8243=ORIENTED_EDGE('',*,*,#6413,.T.);
#8244=ORIENTED_EDGE('',*,*,#6388,.F.);
#8245=ORIENTED_EDGE('',*,*,#6414,.T.);
#8246=ORIENTED_EDGE('',*,*,#6249,.T.);
#8247=ORIENTED_EDGE('',*,*,#6415,.T.);
#8248=ORIENTED_EDGE('',*,*,#6416,.T.);
#8249=ORIENTED_EDGE('',*,*,#6410,.F.);
#8250=ORIENTED_EDGE('',*,*,#6417,.F.);
#8251=ORIENTED_EDGE('',*,*,#6418,.F.);
#8252=ORIENTED_EDGE('',*,*,#6419,.T.);
#8253=ORIENTED_EDGE('',*,*,#6417,.T.);
#8254=ORIENTED_EDGE('',*,*,#6409,.F.);
#8255=ORIENTED_EDGE('',*,*,#6369,.T.);
#8256=ORIENTED_EDGE('',*,*,#6420,.T.);
#8257=ORIENTED_EDGE('',*,*,#6421,.T.);
#8258=ORIENTED_EDGE('',*,*,#6422,.T.);
#8259=ORIENTED_EDGE('',*,*,#6418,.T.);
#8260=ORIENTED_EDGE('',*,*,#6408,.F.);
#8261=ORIENTED_EDGE('',*,*,#6406,.F.);
#8262=ORIENTED_EDGE('',*,*,#6403,.F.);
#8263=ORIENTED_EDGE('',*,*,#6423,.T.);
#8264=ORIENTED_EDGE('',*,*,#6424,.T.);
#8265=ORIENTED_EDGE('',*,*,#6425,.T.);
#8266=ORIENTED_EDGE('',*,*,#6426,.T.);
#8267=ORIENTED_EDGE('',*,*,#6251,.T.);
#8268=ORIENTED_EDGE('',*,*,#6366,.F.);
#8269=ORIENTED_EDGE('',*,*,#6427,.T.);
#8270=ORIENTED_EDGE('',*,*,#6271,.T.);
#8271=ORIENTED_EDGE('',*,*,#6428,.T.);
#8272=ORIENTED_EDGE('',*,*,#6429,.T.);
#8273=ORIENTED_EDGE('',*,*,#6430,.T.);
#8274=ORIENTED_EDGE('',*,*,#6420,.F.);
#8275=ORIENTED_EDGE('',*,*,#6368,.F.);
#8276=ORIENTED_EDGE('',*,*,#6430,.F.);
#8277=ORIENTED_EDGE('',*,*,#6431,.T.);
#8278=ORIENTED_EDGE('',*,*,#6432,.T.);
#8279=ORIENTED_EDGE('',*,*,#6421,.F.);
#8280=ORIENTED_EDGE('',*,*,#6282,.T.);
#8281=ORIENTED_EDGE('',*,*,#6433,.T.);
#8282=ORIENTED_EDGE('',*,*,#6415,.F.);
#8283=ORIENTED_EDGE('',*,*,#6419,.F.);
#8284=ORIENTED_EDGE('',*,*,#6422,.F.);
#8285=ORIENTED_EDGE('',*,*,#6432,.F.);
#8286=ORIENTED_EDGE('',*,*,#6434,.T.);
#8287=ORIENTED_EDGE('',*,*,#6435,.T.);
#8288=ORIENTED_EDGE('',*,*,#6436,.T.);
#8289=ORIENTED_EDGE('',*,*,#6437,.T.);
#8290=ORIENTED_EDGE('',*,*,#6438,.T.);
#8291=ORIENTED_EDGE('',*,*,#6439,.T.);
#8292=ORIENTED_EDGE('',*,*,#6355,.F.);
#8293=ORIENTED_EDGE('',*,*,#6440,.T.);
#8294=ORIENTED_EDGE('',*,*,#6441,.T.);
#8295=ORIENTED_EDGE('',*,*,#6442,.T.);
#8296=ORIENTED_EDGE('',*,*,#6379,.F.);
#8297=ORIENTED_EDGE('',*,*,#6399,.F.);
#8298=ORIENTED_EDGE('',*,*,#6356,.F.);
#8299=ORIENTED_EDGE('',*,*,#6443,.F.);
#8300=ORIENTED_EDGE('',*,*,#6375,.F.);
#8301=ORIENTED_EDGE('',*,*,#6395,.F.);
#8302=ORIENTED_EDGE('',*,*,#6360,.F.);
#8303=ORIENTED_EDGE('',*,*,#6396,.F.);
#8304=ORIENTED_EDGE('',*,*,#6377,.F.);
#8305=ORIENTED_EDGE('',*,*,#6397,.F.);
#8306=ORIENTED_EDGE('',*,*,#6358,.F.);
#8307=ORIENTED_EDGE('',*,*,#6398,.F.);
#8308=ORIENTED_EDGE('',*,*,#6385,.F.);
#8309=ORIENTED_EDGE('',*,*,#6392,.F.);
#8310=ORIENTED_EDGE('',*,*,#6348,.F.);
#8311=ORIENTED_EDGE('',*,*,#6279,.F.);
#8312=ORIENTED_EDGE('',*,*,#6383,.F.);
#8313=ORIENTED_EDGE('',*,*,#6363,.F.);
#8314=ORIENTED_EDGE('',*,*,#6350,.F.);
#8315=ORIENTED_EDGE('',*,*,#6393,.F.);
#8316=ORIENTED_EDGE('',*,*,#6444,.F.);
#8317=ORIENTED_EDGE('',*,*,#6445,.T.);
#8318=ORIENTED_EDGE('',*,*,#6446,.T.);
#8319=ORIENTED_EDGE('',*,*,#6447,.T.);
#8320=ORIENTED_EDGE('',*,*,#6448,.F.);
#8321=ORIENTED_EDGE('',*,*,#6449,.T.);
#8322=ORIENTED_EDGE('',*,*,#6450,.F.);
#8323=ORIENTED_EDGE('',*,*,#6451,.T.);
#8324=ORIENTED_EDGE('',*,*,#6446,.F.);
#8325=ORIENTED_EDGE('',*,*,#6452,.T.);
#8326=ORIENTED_EDGE('',*,*,#6453,.F.);
#8327=ORIENTED_EDGE('',*,*,#6381,.F.);
#8328=ORIENTED_EDGE('',*,*,#6454,.T.);
#8329=ORIENTED_EDGE('',*,*,#6448,.T.);
#8330=ORIENTED_EDGE('',*,*,#6455,.T.);
#8331=ORIENTED_EDGE('',*,*,#6456,.T.);
#8332=ORIENTED_EDGE('',*,*,#6457,.T.);
#8333=ORIENTED_EDGE('',*,*,#6458,.T.);
#8334=ORIENTED_EDGE('',*,*,#6459,.F.);
#8335=ORIENTED_EDGE('',*,*,#6460,.F.);
#8336=ORIENTED_EDGE('',*,*,#6461,.T.);
#8337=ORIENTED_EDGE('',*,*,#6450,.T.);
#8338=ORIENTED_EDGE('',*,*,#6462,.T.);
#8339=ORIENTED_EDGE('',*,*,#6441,.F.);
#8340=ORIENTED_EDGE('',*,*,#6463,.T.);
#8341=ORIENTED_EDGE('',*,*,#6456,.F.);
#8342=ORIENTED_EDGE('',*,*,#6459,.T.);
#8343=ORIENTED_EDGE('',*,*,#6464,.T.);
#8344=ORIENTED_EDGE('',*,*,#6465,.T.);
#8345=ORIENTED_EDGE('',*,*,#6453,.T.);
#8346=ORIENTED_EDGE('',*,*,#6466,.T.);
#8347=ORIENTED_EDGE('',*,*,#6444,.T.);
#8348=ORIENTED_EDGE('',*,*,#6467,.T.);
#8349=ORIENTED_EDGE('',*,*,#6460,.T.);
#8350=ORIENTED_EDGE('',*,*,#6155,.T.);
#8351=ORIENTED_EDGE('',*,*,#6244,.F.);
#8352=ORIENTED_EDGE('',*,*,#6143,.T.);
#8353=ORIENTED_EDGE('',*,*,#6247,.F.);
#8354=ORIENTED_EDGE('',*,*,#6152,.T.);
#8355=ORIENTED_EDGE('',*,*,#6241,.F.);
#8356=ORIENTED_EDGE('',*,*,#6331,.T.);
#8357=ORIENTED_EDGE('',*,*,#6468,.T.);
#8358=ORIENTED_EDGE('',*,*,#6469,.F.);
#8359=ORIENTED_EDGE('',*,*,#6470,.T.);
#8360=ORIENTED_EDGE('',*,*,#6471,.F.);
#8361=ORIENTED_EDGE('',*,*,#6157,.T.);
#8362=ORIENTED_EDGE('',*,*,#6333,.T.);
#8363=ORIENTED_EDGE('',*,*,#6472,.T.);
#8364=ORIENTED_EDGE('',*,*,#6473,.F.);
#8365=ORIENTED_EDGE('',*,*,#6474,.T.);
#8366=ORIENTED_EDGE('',*,*,#6336,.T.);
#8367=ORIENTED_EDGE('',*,*,#6290,.T.);
#8368=ORIENTED_EDGE('',*,*,#6475,.F.);
#8369=ORIENTED_EDGE('',*,*,#6476,.T.);
#8370=ORIENTED_EDGE('',*,*,#6338,.T.);
#8371=ORIENTED_EDGE('',*,*,#6477,.T.);
#8372=ORIENTED_EDGE('',*,*,#6265,.T.);
#8373=ORIENTED_EDGE('',*,*,#6478,.T.);
#8374=ORIENTED_EDGE('',*,*,#6479,.T.);
#8375=ORIENTED_EDGE('',*,*,#6480,.T.);
#8376=ORIENTED_EDGE('',*,*,#6299,.T.);
#8377=ORIENTED_EDGE('',*,*,#6481,.T.);
#8378=ORIENTED_EDGE('',*,*,#6475,.T.);
#8379=ORIENTED_EDGE('',*,*,#6482,.T.);
#8380=ORIENTED_EDGE('',*,*,#6473,.T.);
#8381=ORIENTED_EDGE('',*,*,#6289,.T.);
#8382=ORIENTED_EDGE('',*,*,#6177,.T.);
#8383=ORIENTED_EDGE('',*,*,#6287,.T.);
#8384=ORIENTED_EDGE('',*,*,#6483,.T.);
#8385=ORIENTED_EDGE('',*,*,#6484,.T.);
#8386=ORIENTED_EDGE('',*,*,#6158,.T.);
#8387=ORIENTED_EDGE('',*,*,#6471,.T.);
#8388=ORIENTED_EDGE('',*,*,#6485,.T.);
#8389=ORIENTED_EDGE('',*,*,#6469,.T.);
#8390=ORIENTED_EDGE('',*,*,#6486,.T.);
#8391=ORIENTED_EDGE('',*,*,#6174,.T.);
#8392=ORIENTED_EDGE('',*,*,#6171,.T.);
#8393=ORIENTED_EDGE('',*,*,#6191,.T.);
#8394=ORIENTED_EDGE('',*,*,#6223,.F.);
#8395=ORIENTED_EDGE('',*,*,#6212,.F.);
#8396=ORIENTED_EDGE('',*,*,#6340,.T.);
#8397=ORIENTED_EDGE('',*,*,#6487,.T.);
#8398=ORIENTED_EDGE('',*,*,#6161,.T.);
#8399=ORIENTED_EDGE('',*,*,#6488,.T.);
#8400=ORIENTED_EDGE('',*,*,#6255,.F.);
#8401=ORIENTED_EDGE('',*,*,#6489,.F.);
#8402=ORIENTED_EDGE('',*,*,#6203,.T.);
#8403=ORIENTED_EDGE('',*,*,#6490,.F.);
#8404=ORIENTED_EDGE('',*,*,#6491,.T.);
#8405=ORIENTED_EDGE('',*,*,#6492,.T.);
#8406=ORIENTED_EDGE('',*,*,#6260,.F.);
#8407=ORIENTED_EDGE('',*,*,#6493,.T.);
#8408=ORIENTED_EDGE('',*,*,#6315,.F.);
#8409=ORIENTED_EDGE('',*,*,#6309,.F.);
#8410=ORIENTED_EDGE('',*,*,#6303,.F.);
#8411=ORIENTED_EDGE('',*,*,#6219,.F.);
#8412=ORIENTED_EDGE('',*,*,#6494,.T.);
#8413=ORIENTED_EDGE('',*,*,#6495,.T.);
#8414=ORIENTED_EDGE('',*,*,#6320,.F.);
#8415=ORIENTED_EDGE('',*,*,#6496,.T.);
#8416=ORIENTED_EDGE('',*,*,#6267,.F.);
#8417=ORIENTED_EDGE('',*,*,#6206,.T.);
#8418=ORIENTED_EDGE('',*,*,#6497,.T.);
#8419=ORIENTED_EDGE('',*,*,#6221,.T.);
#8420=ORIENTED_EDGE('',*,*,#6308,.F.);
#8421=ORIENTED_EDGE('',*,*,#6313,.F.);
#8422=ORIENTED_EDGE('',*,*,#6498,.T.);
#8423=ORIENTED_EDGE('',*,*,#6204,.T.);
#8424=ORIENTED_EDGE('',*,*,#6489,.T.);
#8425=ORIENTED_EDGE('',*,*,#6499,.T.);
#8426=ORIENTED_EDGE('',*,*,#6208,.T.);
#8427=ORIENTED_EDGE('',*,*,#6257,.F.);
#8428=ORIENTED_EDGE('',*,*,#6339,.F.);
#8429=ORIENTED_EDGE('',*,*,#6476,.F.);
#8430=ORIENTED_EDGE('',*,*,#6481,.F.);
#8431=ORIENTED_EDGE('',*,*,#6302,.F.);
#8432=ORIENTED_EDGE('',*,*,#6337,.F.);
#8433=ORIENTED_EDGE('',*,*,#6474,.F.);
#8434=ORIENTED_EDGE('',*,*,#6482,.F.);
#8435=ORIENTED_EDGE('',*,*,#6477,.F.);
#8436=ORIENTED_EDGE('',*,*,#6330,.F.);
#8437=ORIENTED_EDGE('',*,*,#6266,.F.);
#8438=ORIENTED_EDGE('',*,*,#6486,.F.);
#8439=ORIENTED_EDGE('',*,*,#6468,.F.);
#8440=ORIENTED_EDGE('',*,*,#6332,.F.);
#8441=ORIENTED_EDGE('',*,*,#6470,.F.);
#8442=ORIENTED_EDGE('',*,*,#6485,.F.);
#8443=ORIENTED_EDGE('',*,*,#6472,.F.);
#8444=ORIENTED_EDGE('',*,*,#6500,.T.);
#8445=ORIENTED_EDGE('',*,*,#6501,.T.);
#8446=ORIENTED_EDGE('',*,*,#6502,.F.);
#8447=ORIENTED_EDGE('',*,*,#6503,.T.);
#8448=ORIENTED_EDGE('',*,*,#6293,.F.);
#8449=ORIENTED_EDGE('',*,*,#6504,.T.);
#8450=ORIENTED_EDGE('',*,*,#6505,.T.);
#8451=ORIENTED_EDGE('',*,*,#6502,.T.);
#8452=ORIENTED_EDGE('',*,*,#6506,.T.);
#8453=ORIENTED_EDGE('',*,*,#6285,.T.);
#8454=ORIENTED_EDGE('',*,*,#6507,.T.);
#8455=ORIENTED_EDGE('',*,*,#6297,.F.);
#8456=ORIENTED_EDGE('',*,*,#6508,.T.);
#8457=ORIENTED_EDGE('',*,*,#6509,.T.);
#8458=ORIENTED_EDGE('',*,*,#6510,.T.);
#8459=ORIENTED_EDGE('',*,*,#6511,.T.);
#8460=ORIENTED_EDGE('',*,*,#6512,.T.);
#8461=ORIENTED_EDGE('',*,*,#6295,.F.);
#8462=ORIENTED_EDGE('',*,*,#6513,.T.);
#8463=ORIENTED_EDGE('',*,*,#6334,.F.);
#8464=ORIENTED_EDGE('',*,*,#6160,.F.);
#8465=ORIENTED_EDGE('',*,*,#6514,.T.);
#8466=ORIENTED_EDGE('',*,*,#6503,.F.);
#8467=ORIENTED_EDGE('',*,*,#6505,.F.);
#8468=ORIENTED_EDGE('',*,*,#6515,.T.);
#8469=ORIENTED_EDGE('',*,*,#6509,.F.);
#8470=ORIENTED_EDGE('',*,*,#6516,.T.);
#8471=ORIENTED_EDGE('',*,*,#6511,.F.);
#8472=ORIENTED_EDGE('',*,*,#6149,.T.);
#8473=ORIENTED_EDGE('',*,*,#6229,.T.);
#8474=ORIENTED_EDGE('',*,*,#6140,.T.);
#8475=ORIENTED_EDGE('',*,*,#6232,.T.);
#8476=ORIENTED_EDGE('',*,*,#6146,.T.);
#8477=ORIENTED_EDGE('',*,*,#6226,.T.);
#8478=ORIENTED_EDGE('',*,*,#6391,.T.);
#8479=ORIENTED_EDGE('',*,*,#6517,.T.);
#8480=ORIENTED_EDGE('',*,*,#6436,.F.);
#8481=ORIENTED_EDGE('',*,*,#6518,.T.);
#8482=ORIENTED_EDGE('',*,*,#6519,.F.);
#8483=ORIENTED_EDGE('',*,*,#6520,.T.);
#8484=ORIENTED_EDGE('',*,*,#6521,.T.);
#8485=ORIENTED_EDGE('',*,*,#6522,.T.);
#8486=ORIENTED_EDGE('',*,*,#6490,.T.);
#8487=ORIENTED_EDGE('',*,*,#6202,.T.);
#8488=ORIENTED_EDGE('',*,*,#6342,.F.);
#8489=ORIENTED_EDGE('',*,*,#6523,.T.);
#8490=ORIENTED_EDGE('',*,*,#6524,.F.);
#8491=ORIENTED_EDGE('',*,*,#6525,.T.);
#8492=ORIENTED_EDGE('',*,*,#6526,.T.);
#8493=ORIENTED_EDGE('',*,*,#6527,.T.);
#8494=ORIENTED_EDGE('',*,*,#6526,.F.);
#8495=ORIENTED_EDGE('',*,*,#6528,.T.);
#8496=ORIENTED_EDGE('',*,*,#6529,.T.);
#8497=ORIENTED_EDGE('',*,*,#6530,.T.);
#8498=ORIENTED_EDGE('',*,*,#6521,.F.);
#8499=ORIENTED_EDGE('',*,*,#6531,.T.);
#8500=ORIENTED_EDGE('',*,*,#6532,.T.);
#8501=ORIENTED_EDGE('',*,*,#6533,.T.);
#8502=ORIENTED_EDGE('',*,*,#6534,.T.);
#8503=ORIENTED_EDGE('',*,*,#6535,.T.);
#8504=ORIENTED_EDGE('',*,*,#6524,.T.);
#8505=ORIENTED_EDGE('',*,*,#6536,.T.);
#8506=ORIENTED_EDGE('',*,*,#6537,.T.);
#8507=ORIENTED_EDGE('',*,*,#6538,.T.);
#8508=ORIENTED_EDGE('',*,*,#6519,.T.);
#8509=ORIENTED_EDGE('',*,*,#6539,.T.);
#8510=ORIENTED_EDGE('',*,*,#6516,.F.);
#8511=ORIENTED_EDGE('',*,*,#6508,.F.);
#8512=ORIENTED_EDGE('',*,*,#6296,.F.);
#8513=ORIENTED_EDGE('',*,*,#6512,.F.);
#8514=ORIENTED_EDGE('',*,*,#6515,.F.);
#8515=ORIENTED_EDGE('',*,*,#6504,.F.);
#8516=ORIENTED_EDGE('',*,*,#6298,.F.);
#8517=ORIENTED_EDGE('',*,*,#6510,.F.);
#8518=ORIENTED_EDGE('',*,*,#6466,.F.);
#8519=ORIENTED_EDGE('',*,*,#6455,.F.);
#8520=ORIENTED_EDGE('',*,*,#6452,.F.);
#8521=ORIENTED_EDGE('',*,*,#6445,.F.);
#8522=ORIENTED_EDGE('',*,*,#6467,.F.);
#8523=ORIENTED_EDGE('',*,*,#6447,.F.);
#8524=ORIENTED_EDGE('',*,*,#6451,.F.);
#8525=ORIENTED_EDGE('',*,*,#6461,.F.);
#8526=ORIENTED_EDGE('',*,*,#6261,.F.);
#8527=ORIENTED_EDGE('',*,*,#6495,.F.);
#8528=ORIENTED_EDGE('',*,*,#6540,.F.);
#8529=ORIENTED_EDGE('',*,*,#6491,.F.);
#8530=ORIENTED_EDGE('',*,*,#6523,.F.);
#8531=ORIENTED_EDGE('',*,*,#6540,.T.);
#8532=ORIENTED_EDGE('',*,*,#6494,.F.);
#8533=ORIENTED_EDGE('',*,*,#6209,.F.);
#8534=ORIENTED_EDGE('',*,*,#6499,.F.);
#8535=ORIENTED_EDGE('',*,*,#6492,.F.);
#8536=ORIENTED_EDGE('',*,*,#6211,.T.);
#8537=ORIENTED_EDGE('',*,*,#6497,.F.);
#8538=ORIENTED_EDGE('',*,*,#6205,.F.);
#8539=ORIENTED_EDGE('',*,*,#6498,.F.);
#8540=ORIENTED_EDGE('',*,*,#6518,.F.);
#8541=ORIENTED_EDGE('',*,*,#6439,.F.);
#8542=ORIENTED_EDGE('',*,*,#6541,.F.);
#8543=ORIENTED_EDGE('',*,*,#6428,.F.);
#8544=ORIENTED_EDGE('',*,*,#6275,.F.);
#8545=ORIENTED_EDGE('',*,*,#6283,.F.);
#8546=ORIENTED_EDGE('',*,*,#6435,.F.);
#8547=ORIENTED_EDGE('',*,*,#6542,.F.);
#8548=ORIENTED_EDGE('',*,*,#6437,.F.);
#8549=ORIENTED_EDGE('',*,*,#6517,.F.);
#8550=ORIENTED_EDGE('',*,*,#6543,.F.);
#8551=ORIENTED_EDGE('',*,*,#6438,.F.);
#8552=ORIENTED_EDGE('',*,*,#6544,.F.);
#8553=ORIENTED_EDGE('',*,*,#6426,.F.);
#8554=ORIENTED_EDGE('',*,*,#6541,.T.);
#8555=ORIENTED_EDGE('',*,*,#6543,.T.);
#8556=ORIENTED_EDGE('',*,*,#6545,.F.);
#8557=ORIENTED_EDGE('',*,*,#6544,.T.);
#8558=ORIENTED_EDGE('',*,*,#6542,.T.);
#8559=ORIENTED_EDGE('',*,*,#6546,.F.);
#8560=ORIENTED_EDGE('',*,*,#6545,.T.);
#8561=ORIENTED_EDGE('',*,*,#6425,.F.);
#8562=ORIENTED_EDGE('',*,*,#6547,.F.);
#8563=ORIENTED_EDGE('',*,*,#6429,.F.);
#8564=ORIENTED_EDGE('',*,*,#6546,.T.);
#8565=ORIENTED_EDGE('',*,*,#6434,.F.);
#8566=ORIENTED_EDGE('',*,*,#6548,.F.);
#8567=ORIENTED_EDGE('',*,*,#6423,.F.);
#8568=ORIENTED_EDGE('',*,*,#6547,.T.);
#8569=ORIENTED_EDGE('',*,*,#6424,.F.);
#8570=ORIENTED_EDGE('',*,*,#6548,.T.);
#8571=ORIENTED_EDGE('',*,*,#6431,.F.);
#8572=ORIENTED_EDGE('',*,*,#6500,.F.);
#8573=ORIENTED_EDGE('',*,*,#6514,.F.);
#8574=ORIENTED_EDGE('',*,*,#6159,.T.);
#8575=ORIENTED_EDGE('',*,*,#6484,.F.);
#8576=ORIENTED_EDGE('',*,*,#6549,.T.);
#8577=ORIENTED_EDGE('',*,*,#6458,.F.);
#8578=ORIENTED_EDGE('',*,*,#6550,.T.);
#8579=ORIENTED_EDGE('',*,*,#6353,.F.);
#8580=ORIENTED_EDGE('',*,*,#6551,.T.);
#8581=ORIENTED_EDGE('',*,*,#6464,.F.);
#8582=ORIENTED_EDGE('',*,*,#6531,.F.);
#8583=ORIENTED_EDGE('',*,*,#6520,.F.);
#8584=ORIENTED_EDGE('',*,*,#6538,.F.);
#8585=ORIENTED_EDGE('',*,*,#6552,.T.);
#8586=ORIENTED_EDGE('',*,*,#6479,.F.);
#8587=ORIENTED_EDGE('',*,*,#6553,.T.);
#8588=ORIENTED_EDGE('',*,*,#6530,.F.);
#8589=ORIENTED_EDGE('',*,*,#6554,.T.);
#8590=ORIENTED_EDGE('',*,*,#6346,.F.);
#8591=ORIENTED_EDGE('',*,*,#6555,.T.);
#8592=ORIENTED_EDGE('',*,*,#6539,.F.);
#8593=ORIENTED_EDGE('',*,*,#6522,.F.);
#8594=ORIENTED_EDGE('',*,*,#6323,.F.);
#8595=ORIENTED_EDGE('',*,*,#6316,.F.);
#8596=ORIENTED_EDGE('',*,*,#6493,.F.);
#8597=ORIENTED_EDGE('',*,*,#6259,.F.);
#8598=ORIENTED_EDGE('',*,*,#6496,.F.);
#8599=ORIENTED_EDGE('',*,*,#6319,.F.);
#8600=ORIENTED_EDGE('',*,*,#6326,.F.);
#8601=ORIENTED_EDGE('',*,*,#6268,.F.);
#8602=ORIENTED_EDGE('',*,*,#6462,.F.);
#8603=ORIENTED_EDGE('',*,*,#6449,.F.);
#8604=ORIENTED_EDGE('',*,*,#6454,.F.);
#8605=ORIENTED_EDGE('',*,*,#6380,.F.);
#8606=ORIENTED_EDGE('',*,*,#6442,.F.);
#8607=ORIENTED_EDGE('',*,*,#6292,.F.);
#8608=ORIENTED_EDGE('',*,*,#6335,.F.);
#8609=ORIENTED_EDGE('',*,*,#6513,.F.);
#8610=ORIENTED_EDGE('',*,*,#6294,.F.);
#8611=ORIENTED_EDGE('',*,*,#6507,.F.);
#8612=ORIENTED_EDGE('',*,*,#6433,.F.);
#8613=ORIENTED_EDGE('',*,*,#6281,.F.);
#8614=ORIENTED_EDGE('',*,*,#6411,.F.);
#8615=ORIENTED_EDGE('',*,*,#6416,.F.);
#8616=ORIENTED_EDGE('',*,*,#6402,.F.);
#8617=ORIENTED_EDGE('',*,*,#6272,.F.);
#8618=ORIENTED_EDGE('',*,*,#6427,.F.);
#8619=ORIENTED_EDGE('',*,*,#6365,.F.);
#8620=ORIENTED_EDGE('',*,*,#6183,.T.);
#8621=ORIENTED_EDGE('',*,*,#6443,.T.);
#8622=ORIENTED_EDGE('',*,*,#6186,.T.);
#8623=ORIENTED_EDGE('',*,*,#6235,.F.);
#8624=ORIENTED_EDGE('',*,*,#6181,.T.);
#8625=ORIENTED_EDGE('',*,*,#6217,.F.);
#8626=ORIENTED_EDGE('',*,*,#6178,.T.);
#8627=ORIENTED_EDGE('',*,*,#6288,.T.);
#8628=ORIENTED_EDGE('',*,*,#6341,.F.);
#8629=ORIENTED_EDGE('',*,*,#6488,.F.);
#8630=ORIENTED_EDGE('',*,*,#6164,.F.);
#8631=ORIENTED_EDGE('',*,*,#6322,.F.);
#8632=ORIENTED_EDGE('',*,*,#6343,.F.);
#8633=ORIENTED_EDGE('',*,*,#6324,.F.);
#8634=ORIENTED_EDGE('',*,*,#6162,.T.);
#8635=ORIENTED_EDGE('',*,*,#6487,.F.);
#8636=ORIENTED_EDGE('',*,*,#6387,.F.);
#8637=ORIENTED_EDGE('',*,*,#6401,.F.);
#8638=ORIENTED_EDGE('',*,*,#6556,.F.);
#8639=ORIENTED_EDGE('',*,*,#6414,.F.);
#8640=ORIENTED_EDGE('',*,*,#6556,.T.);
#8641=ORIENTED_EDGE('',*,*,#6405,.F.);
#8642=ORIENTED_EDGE('',*,*,#6557,.F.);
#8643=ORIENTED_EDGE('',*,*,#6412,.F.);
#8644=ORIENTED_EDGE('',*,*,#6389,.F.);
#8645=ORIENTED_EDGE('',*,*,#6413,.F.);
#8646=ORIENTED_EDGE('',*,*,#6557,.T.);
#8647=ORIENTED_EDGE('',*,*,#6407,.F.);
#8648=ORIENTED_EDGE('',*,*,#6529,.F.);
#8649=ORIENTED_EDGE('',*,*,#6558,.T.);
#8650=ORIENTED_EDGE('',*,*,#6371,.F.);
#8651=ORIENTED_EDGE('',*,*,#6277,.F.);
#8652=ORIENTED_EDGE('',*,*,#6347,.F.);
#8653=ORIENTED_EDGE('',*,*,#6554,.F.);
#8654=ORIENTED_EDGE('',*,*,#6329,.F.);
#8655=ORIENTED_EDGE('',*,*,#6559,.T.);
#8656=ORIENTED_EDGE('',*,*,#6532,.F.);
#8657=ORIENTED_EDGE('',*,*,#6553,.F.);
#8658=ORIENTED_EDGE('',*,*,#6478,.F.);
#8659=ORIENTED_EDGE('',*,*,#6264,.F.);
#8660=ORIENTED_EDGE('',*,*,#6537,.F.);
#8661=ORIENTED_EDGE('',*,*,#6560,.T.);
#8662=ORIENTED_EDGE('',*,*,#6327,.F.);
#8663=ORIENTED_EDGE('',*,*,#6300,.F.);
#8664=ORIENTED_EDGE('',*,*,#6480,.F.);
#8665=ORIENTED_EDGE('',*,*,#6552,.F.);
#8666=ORIENTED_EDGE('',*,*,#6373,.F.);
#8667=ORIENTED_EDGE('',*,*,#6561,.T.);
#8668=ORIENTED_EDGE('',*,*,#6534,.F.);
#8669=ORIENTED_EDGE('',*,*,#6555,.F.);
#8670=ORIENTED_EDGE('',*,*,#6345,.F.);
#8671=ORIENTED_EDGE('',*,*,#6394,.F.);
#8672=ORIENTED_EDGE('',*,*,#6352,.F.);
#8673=ORIENTED_EDGE('',*,*,#6362,.F.);
#8674=ORIENTED_EDGE('',*,*,#6382,.F.);
#8675=ORIENTED_EDGE('',*,*,#6465,.F.);
#8676=ORIENTED_EDGE('',*,*,#6551,.F.);
#8677=ORIENTED_EDGE('',*,*,#6506,.F.);
#8678=ORIENTED_EDGE('',*,*,#6501,.F.);
#8679=ORIENTED_EDGE('',*,*,#6549,.F.);
#8680=ORIENTED_EDGE('',*,*,#6483,.F.);
#8681=ORIENTED_EDGE('',*,*,#6286,.F.);
#8682=ORIENTED_EDGE('',*,*,#6463,.F.);
#8683=ORIENTED_EDGE('',*,*,#6440,.F.);
#8684=ORIENTED_EDGE('',*,*,#6354,.F.);
#8685=ORIENTED_EDGE('',*,*,#6550,.F.);
#8686=ORIENTED_EDGE('',*,*,#6457,.F.);
#8687=ORIENTED_EDGE('',*,*,#6528,.F.);
#8688=ORIENTED_EDGE('',*,*,#6525,.F.);
#8689=ORIENTED_EDGE('',*,*,#6535,.F.);
#8690=ORIENTED_EDGE('',*,*,#6561,.F.);
#8691=ORIENTED_EDGE('',*,*,#6372,.F.);
#8692=ORIENTED_EDGE('',*,*,#6558,.F.);
#8693=ORIENTED_EDGE('',*,*,#6559,.F.);
#8694=ORIENTED_EDGE('',*,*,#6328,.F.);
#8695=ORIENTED_EDGE('',*,*,#6560,.F.);
#8696=ORIENTED_EDGE('',*,*,#6536,.F.);
#8697=ORIENTED_EDGE('',*,*,#6527,.F.);
#8698=ORIENTED_EDGE('',*,*,#6533,.F.);
#11277=CONICAL_SURFACE('',#12300,13.,0.785398163397443);
#11278=CONICAL_SURFACE('',#12303,12.4000000000001,0.785398163397443);
#11279=CONICAL_SURFACE('',#12306,13.,0.785398163397454);
#11280=CONICAL_SURFACE('',#12309,16.,0.785398163397466);
#11281=CONICAL_SURFACE('',#12312,12.4000000000001,0.785398163397443);
#11282=CONICAL_SURFACE('',#12315,15.4,0.785398163397495);
#11329=ADVANCED_FACE('',(#1247),#11277,.T.);
#11330=ADVANCED_FACE('',(#1248),#11278,.T.);
#11331=ADVANCED_FACE('',(#1249),#11279,.T.);
#11332=ADVANCED_FACE('',(#1250),#11280,.T.);
#11333=ADVANCED_FACE('',(#1251),#11281,.T.);
#11334=ADVANCED_FACE('',(#1252),#11282,.T.);
#11335=ADVANCED_FACE('',(#1253),#975,.F.);
#11336=ADVANCED_FACE('',(#1254),#811,.T.);
#11337=ADVANCED_FACE('',(#1255),#812,.F.);
#11338=ADVANCED_FACE('',(#1256),#813,.F.);
#11339=ADVANCED_FACE('',(#1257),#814,.F.);
#11340=ADVANCED_FACE('',(#1258),#815,.F.);
#11341=ADVANCED_FACE('',(#1259),#816,.F.);
#11342=ADVANCED_FACE('',(#1260),#817,.F.);
#11343=ADVANCED_FACE('',(#1261),#818,.F.);
#11344=ADVANCED_FACE('',(#1262),#819,.F.);
#11345=ADVANCED_FACE('',(#1263),#820,.F.);
#11346=ADVANCED_FACE('',(#1264),#821,.F.);
#11347=ADVANCED_FACE('',(#1265),#976,.F.);
#11348=ADVANCED_FACE('',(#1266),#822,.F.);
#11349=ADVANCED_FACE('',(#1267),#977,.F.);
#11350=ADVANCED_FACE('',(#1268),#978,.T.);
#11351=ADVANCED_FACE('',(#1269),#979,.T.);
#11352=ADVANCED_FACE('',(#1270),#980,.T.);
#11353=ADVANCED_FACE('',(#1271),#981,.F.);
#11354=ADVANCED_FACE('',(#1272),#982,.T.);
#11355=ADVANCED_FACE('',(#1273),#983,.F.);
#11356=ADVANCED_FACE('',(#1274),#984,.F.);
#11357=ADVANCED_FACE('',(#1275),#985,.F.);
#11358=ADVANCED_FACE('',(#1276),#986,.T.);
#11359=ADVANCED_FACE('',(#1277),#987,.T.);
#11360=ADVANCED_FACE('',(#1278),#988,.T.);
#11361=ADVANCED_FACE('',(#1279),#989,.T.);
#11362=ADVANCED_FACE('',(#1280),#990,.F.);
#11363=ADVANCED_FACE('',(#1281),#991,.F.);
#11364=ADVANCED_FACE('',(#1282),#992,.F.);
#11365=ADVANCED_FACE('',(#1283),#993,.T.);
#11366=ADVANCED_FACE('',(#1284),#994,.F.);
#11367=ADVANCED_FACE('',(#1285),#995,.T.);
#11368=ADVANCED_FACE('',(#1286),#996,.F.);
#11369=ADVANCED_FACE('',(#1287),#448,.T.);
#11370=ADVANCED_FACE('',(#1288),#449,.T.);
#11371=ADVANCED_FACE('',(#1289),#450,.T.);
#11372=ADVANCED_FACE('',(#1290),#451,.F.);
#11373=ADVANCED_FACE('',(#1291),#452,.F.);
#11374=ADVANCED_FACE('',(#1292),#453,.F.);
#11375=ADVANCED_FACE('',(#1293),#997,.T.);
#11376=ADVANCED_FACE('',(#1294),#454,.F.);
#11377=ADVANCED_FACE('',(#1295),#455,.T.);
#11378=ADVANCED_FACE('',(#1296),#456,.T.);
#11379=ADVANCED_FACE('',(#1297),#998,.F.);
#11380=ADVANCED_FACE('',(#1298),#999,.F.);
#11381=ADVANCED_FACE('',(#1299),#457,.T.);
#11382=ADVANCED_FACE('',(#1300),#458,.T.);
#11383=ADVANCED_FACE('',(#1301),#459,.F.);
#11384=ADVANCED_FACE('',(#1302),#460,.F.);
#11385=ADVANCED_FACE('',(#1303,#335,#336,#337,#338,#339),#461,.T.);
#11386=ADVANCED_FACE('',(#1304,#340,#341,#342),#462,.F.);
#11387=ADVANCED_FACE('',(#1305),#463,.F.);
#11388=ADVANCED_FACE('',(#1306),#464,.F.);
#11389=ADVANCED_FACE('',(#1307),#1000,.F.);
#11390=ADVANCED_FACE('',(#1308,#343,#344,#345,#346,#347),#465,.T.);
#11391=ADVANCED_FACE('',(#1309),#466,.F.);
#11392=ADVANCED_FACE('',(#1310),#467,.F.);
#11393=ADVANCED_FACE('',(#1311),#468,.F.);
#11394=ADVANCED_FACE('',(#1312),#469,.F.);
#11395=ADVANCED_FACE('',(#1313,#348),#470,.T.);
#11396=ADVANCED_FACE('',(#1314),#471,.T.);
#11397=ADVANCED_FACE('',(#1315),#1001,.T.);
#11398=ADVANCED_FACE('',(#1316),#472,.T.);
#11399=ADVANCED_FACE('',(#1317,#349),#473,.F.);
#11400=ADVANCED_FACE('',(#1318),#474,.F.);
#11401=ADVANCED_FACE('',(#1319),#1002,.F.);
#11402=ADVANCED_FACE('',(#1320),#475,.F.);
#11403=ADVANCED_FACE('',(#1321,#350),#476,.T.);
#11404=ADVANCED_FACE('',(#1322),#477,.F.);
#11405=ADVANCED_FACE('',(#1323),#1003,.F.);
#11406=ADVANCED_FACE('',(#1324),#478,.F.);
#11407=ADVANCED_FACE('',(#1325),#479,.F.);
#11408=ADVANCED_FACE('',(#1326),#1004,.T.);
#11409=ADVANCED_FACE('',(#1327),#1005,.T.);
#11410=ADVANCED_FACE('',(#1328),#1006,.T.);
#11411=ADVANCED_FACE('',(#1329),#1007,.T.);
#11412=ADVANCED_FACE('',(#1330),#1008,.T.);
#11413=ADVANCED_FACE('',(#1331),#480,.F.);
#11414=ADVANCED_FACE('',(#1332),#481,.F.);
#11415=ADVANCED_FACE('',(#1333),#482,.F.);
#11416=ADVANCED_FACE('',(#1334),#483,.F.);
#11417=ADVANCED_FACE('',(#1335),#484,.F.);
#11418=ADVANCED_FACE('',(#1336),#485,.T.);
#11419=ADVANCED_FACE('',(#1337,#351),#486,.T.);
#11420=ADVANCED_FACE('',(#1338,#352),#487,.T.);
#11421=ADVANCED_FACE('',(#1339,#353),#488,.T.);
#11422=ADVANCED_FACE('',(#1340),#489,.T.);
#11423=ADVANCED_FACE('',(#1341),#490,.T.);
#11424=ADVANCED_FACE('',(#1342),#491,.T.);
#11425=ADVANCED_FACE('',(#1343),#492,.T.);
#11426=ADVANCED_FACE('',(#1344,#354,#355,#356),#493,.F.);
#11427=ADVANCED_FACE('',(#1345,#357),#494,.T.);
#11428=ADVANCED_FACE('',(#1346,#358),#495,.F.);
#11429=ADVANCED_FACE('',(#1347),#496,.T.);
#11430=ADVANCED_FACE('',(#1348),#497,.T.);
#11431=ADVANCED_FACE('',(#1349),#498,.T.);
#11432=ADVANCED_FACE('',(#1350,#359),#499,.T.);
#11433=ADVANCED_FACE('',(#1351),#1009,.T.);
#11434=ADVANCED_FACE('',(#1352),#1010,.T.);
#11435=ADVANCED_FACE('',(#1353),#1011,.T.);
#11436=ADVANCED_FACE('',(#1354),#1012,.T.);
#11437=ADVANCED_FACE('',(#1355),#500,.T.);
#11438=ADVANCED_FACE('',(#1356),#501,.T.);
#11439=ADVANCED_FACE('',(#1357),#502,.T.);
#11440=ADVANCED_FACE('',(#1358),#503,.T.);
#11441=ADVANCED_FACE('',(#1359),#504,.T.);
#11442=ADVANCED_FACE('',(#1360,#360),#505,.T.);
#11443=ADVANCED_FACE('',(#1361,#361),#506,.T.);
#11444=ADVANCED_FACE('',(#1362,#362),#507,.T.);
#11445=ADVANCED_FACE('',(#1363),#508,.T.);
#11446=ADVANCED_FACE('',(#1364),#509,.T.);
#11447=ADVANCED_FACE('',(#1365),#510,.T.);
#11448=ADVANCED_FACE('',(#1366),#511,.T.);
#11449=ADVANCED_FACE('',(#1367),#512,.F.);
#11450=ADVANCED_FACE('',(#1368),#513,.T.);
#11451=ADVANCED_FACE('',(#1369),#1013,.T.);
#11452=ADVANCED_FACE('',(#1370),#1014,.T.);
#11453=ADVANCED_FACE('',(#1371),#1015,.T.);
#11454=ADVANCED_FACE('',(#1372),#1016,.T.);
#11455=ADVANCED_FACE('',(#1373),#1017,.F.);
#11456=ADVANCED_FACE('',(#1374),#1018,.F.);
#11457=ADVANCED_FACE('',(#1375),#1019,.F.);
#11458=ADVANCED_FACE('',(#1376),#1020,.F.);
#11459=ADVANCED_FACE('',(#1377),#1021,.F.);
#11460=ADVANCED_FACE('',(#1378),#1022,.F.);
#11461=ADVANCED_FACE('',(#1379),#327,.F.);
#11462=ADVANCED_FACE('',(#1380),#328,.F.);
#11463=ADVANCED_FACE('',(#1381),#1023,.F.);
#11464=ADVANCED_FACE('',(#1382),#1024,.F.);
#11465=ADVANCED_FACE('',(#1383),#823,.F.);
#11466=ADVANCED_FACE('',(#1384),#1025,.T.);
#11467=ADVANCED_FACE('',(#1385),#1026,.T.);
#11468=ADVANCED_FACE('',(#1386),#1027,.F.);
#11469=ADVANCED_FACE('',(#1387),#1028,.F.);
#11470=ADVANCED_FACE('',(#1388),#1029,.T.);
#11471=ADVANCED_FACE('',(#1389),#1030,.T.);
#11472=ADVANCED_FACE('',(#1390),#1031,.F.);
#11473=ADVANCED_FACE('',(#1391),#1032,.F.);
#11474=ADVANCED_FACE('',(#1392),#1033,.T.);
#11475=ADVANCED_FACE('',(#1393),#1034,.T.);
#11476=ADVANCED_FACE('',(#1394),#308,.F.);
#11477=ADVANCED_FACE('',(#1395),#309,.F.);
#11478=ADVANCED_FACE('',(#1396),#1035,.T.);
#11479=ADVANCED_FACE('',(#1397),#1036,.T.);
#11480=ADVANCED_FACE('',(#1398),#1037,.T.);
#11481=ADVANCED_FACE('',(#1399),#824,.T.);
#11482=ADVANCED_FACE('',(#1400),#1038,.T.);
#11483=ADVANCED_FACE('',(#1401),#1039,.F.);
#11484=ADVANCED_FACE('',(#1402),#1040,.F.);
#11485=ADVANCED_FACE('',(#1403),#1041,.F.);
#11486=ADVANCED_FACE('',(#1404),#1042,.F.);
#11487=ADVANCED_FACE('',(#1405),#1043,.F.);
#11488=ADVANCED_FACE('',(#1406),#1044,.F.);
#11489=ADVANCED_FACE('',(#1407),#1045,.F.);
#11490=ADVANCED_FACE('',(#1408),#1046,.T.);
#11491=ADVANCED_FACE('',(#1409),#1047,.T.);
#12026=CLOSED_SHELL('',(#11329,#11330,#11331,#11332,#11333,#11334,#11335,
#11336,#11337,#11338,#11339,#11340,#11341,#11342,#11343,#11344,#11345,#11346,
#11347,#11348,#11349,#11350,#11351,#11352,#11353,#11354,#11355,#11356,#11357,
#11358,#11359,#11360,#11361,#11362,#11363,#11364,#11365,#11366,#11367,#11368,
#11369,#11370,#11371,#11372,#11373,#11374,#11375,#11376,#11377,#11378,#11379,
#11380,#11381,#11382,#11383,#11384,#11385,#11386,#11387,#11388,#11389,#11390,
#11391,#11392,#11393,#11394,#11395,#11396,#11397,#11398,#11399,#11400,#11401,
#11402,#11403,#11404,#11405,#11406,#11407,#11408,#11409,#11410,#11411,#11412,
#11413,#11414,#11415,#11416,#11417,#11418,#11419,#11420,#11421,#11422,#11423,
#11424,#11425,#11426,#11427,#11428,#11429,#11430,#11431,#11432,#11433,#11434,
#11435,#11436,#11437,#11438,#11439,#11440,#11441,#11442,#11443,#11444,#11445,
#11446,#11447,#11448,#11449,#11450,#11451,#11452,#11453,#11454,#11455,#11456,
#11457,#11458,#11459,#11460,#11461,#11462,#11463,#11464,#11465,#11466,#11467,
#11468,#11469,#11470,#11471,#11472,#11473,#11474,#11475,#11476,#11477,#11478,
#11479,#11480,#11481,#11482,#11483,#11484,#11485,#11486,#11487,#11488,#11489,
#11490,#11491));
#12299=AXIS2_PLACEMENT_3D('',#17421,#13734,#13735);
#12300=AXIS2_PLACEMENT_3D('',#17422,#13736,#13737);
#12301=AXIS2_PLACEMENT_3D('',#17424,#13738,#13739);
#12302=AXIS2_PLACEMENT_3D('',#17427,#13741,#13742);
#12303=AXIS2_PLACEMENT_3D('',#17428,#13743,#13744);
#12304=AXIS2_PLACEMENT_3D('',#17430,#13745,#13746);
#12305=AXIS2_PLACEMENT_3D('',#17433,#13748,#13749);
#12306=AXIS2_PLACEMENT_3D('',#17434,#13750,#13751);
#12307=AXIS2_PLACEMENT_3D('',#17436,#13752,#13753);
#12308=AXIS2_PLACEMENT_3D('',#17439,#13755,#13756);
#12309=AXIS2_PLACEMENT_3D('',#17440,#13757,#13758);
#12310=AXIS2_PLACEMENT_3D('',#17442,#13759,#13760);
#12311=AXIS2_PLACEMENT_3D('',#17445,#13762,#13763);
#12312=AXIS2_PLACEMENT_3D('',#17446,#13764,#13765);
#12313=AXIS2_PLACEMENT_3D('',#17448,#13766,#13767);
#12314=AXIS2_PLACEMENT_3D('',#17451,#13769,#13770);
#12315=AXIS2_PLACEMENT_3D('',#17452,#13771,#13772);
#12316=AXIS2_PLACEMENT_3D('',#17454,#13773,#13774);
#12317=AXIS2_PLACEMENT_3D('',#17457,#13776,#13777);
#12318=AXIS2_PLACEMENT_3D('',#17458,#13778,#13779);
#12319=AXIS2_PLACEMENT_3D('',#17461,#13780,#13781);
#12320=AXIS2_PLACEMENT_3D('',#17465,#13783,#13784);
#12321=AXIS2_PLACEMENT_3D('',#17480,#13786,#13787);
#12322=AXIS2_PLACEMENT_3D('',#17483,#13788,#13789);
#12323=AXIS2_PLACEMENT_3D('',#17485,#13790,#13791);
#12324=AXIS2_PLACEMENT_3D('',#17487,#13792,#13793);
#12325=AXIS2_PLACEMENT_3D('',#17488,#13794,#13795);
#12326=AXIS2_PLACEMENT_3D('',#17489,#13796,#13797);
#12327=AXIS2_PLACEMENT_3D('',#17491,#13798,#13799);
#12328=AXIS2_PLACEMENT_3D('',#17493,#13800,#13801);
#12329=AXIS2_PLACEMENT_3D('',#17494,#13802,#13803);
#12330=AXIS2_PLACEMENT_3D('',#17495,#13804,#13805);
#12331=AXIS2_PLACEMENT_3D('',#17497,#13806,#13807);
#12332=AXIS2_PLACEMENT_3D('',#17499,#13808,#13809);
#12333=AXIS2_PLACEMENT_3D('',#17500,#13810,#13811);
#12334=AXIS2_PLACEMENT_3D('',#17501,#13812,#13813);
#12335=AXIS2_PLACEMENT_3D('',#17503,#13814,#13815);
#12336=AXIS2_PLACEMENT_3D('',#17505,#13816,#13817);
#12337=AXIS2_PLACEMENT_3D('',#17506,#13818,#13819);
#12338=AXIS2_PLACEMENT_3D('',#17507,#13820,#13821);
#12339=AXIS2_PLACEMENT_3D('',#17509,#13822,#13823);
#12340=AXIS2_PLACEMENT_3D('',#17511,#13824,#13825);
#12341=AXIS2_PLACEMENT_3D('',#17512,#13826,#13827);
#12342=AXIS2_PLACEMENT_3D('',#17513,#13828,#13829);
#12343=AXIS2_PLACEMENT_3D('',#17516,#13830,#13831);
#12344=AXIS2_PLACEMENT_3D('',#17518,#13832,#13833);
#12345=AXIS2_PLACEMENT_3D('',#17520,#13834,#13835);
#12346=AXIS2_PLACEMENT_3D('',#17522,#13836,#13837);
#12347=AXIS2_PLACEMENT_3D('',#17523,#13838,#13839);
#12348=AXIS2_PLACEMENT_3D('',#17524,#13840,#13841);
#12349=AXIS2_PLACEMENT_3D('',#17527,#13842,#13843);
#12350=AXIS2_PLACEMENT_3D('',#17529,#13844,#13845);
#12351=AXIS2_PLACEMENT_3D('',#17531,#13846,#13847);
#12352=AXIS2_PLACEMENT_3D('',#17533,#13848,#13849);
#12353=AXIS2_PLACEMENT_3D('',#17534,#13850,#13851);
#12354=AXIS2_PLACEMENT_3D('',#17535,#13852,#13853);
#12355=AXIS2_PLACEMENT_3D('',#17537,#13854,#13855);
#12356=AXIS2_PLACEMENT_3D('',#17539,#13856,#13857);
#12357=AXIS2_PLACEMENT_3D('',#17541,#13858,#13859);
#12358=AXIS2_PLACEMENT_3D('',#17542,#13860,#13861);
#12359=AXIS2_PLACEMENT_3D('',#17543,#13862,#13863);
#12360=AXIS2_PLACEMENT_3D('',#17545,#13864,#13865);
#12361=AXIS2_PLACEMENT_3D('',#17547,#13866,#13867);
#12362=AXIS2_PLACEMENT_3D('',#17548,#13868,#13869);
#12363=AXIS2_PLACEMENT_3D('',#17549,#13870,#13871);
#12364=AXIS2_PLACEMENT_3D('',#17552,#13872,#13873);
#12365=AXIS2_PLACEMENT_3D('',#17553,#13874,#13875);
#12366=AXIS2_PLACEMENT_3D('',#17555,#13876,#13877);
#12367=AXIS2_PLACEMENT_3D('',#17556,#13878,#13879);
#12368=AXIS2_PLACEMENT_3D('',#17557,#13880,#13881);
#12369=AXIS2_PLACEMENT_3D('',#17560,#13882,#13883);
#12370=AXIS2_PLACEMENT_3D('',#17561,#13884,#13885);
#12371=AXIS2_PLACEMENT_3D('',#17563,#13886,#13887);
#12372=AXIS2_PLACEMENT_3D('',#17564,#13888,#13889);
#12373=AXIS2_PLACEMENT_3D('',#17565,#13890,#13891);
#12374=AXIS2_PLACEMENT_3D('',#17568,#13892,#13893);
#12375=AXIS2_PLACEMENT_3D('',#17572,#13895,#13896);
#12376=AXIS2_PLACEMENT_3D('',#17574,#13897,#13898);
#12377=AXIS2_PLACEMENT_3D('',#17577,#13900,#13901);
#12378=AXIS2_PLACEMENT_3D('',#17578,#13902,#13903);
#12379=AXIS2_PLACEMENT_3D('',#17581,#13904,#13905);
#12380=AXIS2_PLACEMENT_3D('',#17583,#13906,#13907);
#12381=AXIS2_PLACEMENT_3D('',#17585,#13908,#13909);
#12382=AXIS2_PLACEMENT_3D('',#17586,#13910,#13911);
#12383=AXIS2_PLACEMENT_3D('',#17587,#13912,#13913);
#12384=AXIS2_PLACEMENT_3D('',#17589,#13914,#13915);
#12385=AXIS2_PLACEMENT_3D('',#17592,#13917,#13918);
#12386=AXIS2_PLACEMENT_3D('',#17593,#13919,#13920);
#12387=AXIS2_PLACEMENT_3D('',#17595,#13922,#13923);
#12388=AXIS2_PLACEMENT_3D('',#17609,#13925,#13926);
#12389=AXIS2_PLACEMENT_3D('',#17611,#13928,#13929);
#12390=AXIS2_PLACEMENT_3D('',#17615,#13931,#13932);
#12391=AXIS2_PLACEMENT_3D('',#17617,#13934,#13935);
#12392=AXIS2_PLACEMENT_3D('',#17620,#13937,#13938);
#12393=AXIS2_PLACEMENT_3D('',#17621,#13939,#13940);
#12394=AXIS2_PLACEMENT_3D('',#17623,#13941,#13942);
#12395=AXIS2_PLACEMENT_3D('',#17626,#13944,#13945);
#12396=AXIS2_PLACEMENT_3D('',#17627,#13946,#13947);
#12397=AXIS2_PLACEMENT_3D('',#17629,#13948,#13949);
#12398=AXIS2_PLACEMENT_3D('',#17632,#13951,#13952);
#12399=AXIS2_PLACEMENT_3D('',#17633,#13953,#13954);
#12400=AXIS2_PLACEMENT_3D('',#17635,#13955,#13956);
#12401=AXIS2_PLACEMENT_3D('',#17638,#13958,#13959);
#12402=AXIS2_PLACEMENT_3D('',#17639,#13960,#13961);
#12403=AXIS2_PLACEMENT_3D('',#17641,#13963,#13964);
#12404=AXIS2_PLACEMENT_3D('',#17655,#13966,#13967);
#12405=AXIS2_PLACEMENT_3D('',#17657,#13969,#13970);
#12406=AXIS2_PLACEMENT_3D('',#17660,#13972,#13973);
#12407=AXIS2_PLACEMENT_3D('',#17661,#13974,#13975);
#12408=AXIS2_PLACEMENT_3D('',#17663,#13976,#13977);
#12409=AXIS2_PLACEMENT_3D('',#17666,#13979,#13980);
#12410=AXIS2_PLACEMENT_3D('',#17667,#13981,#13982);
#12411=AXIS2_PLACEMENT_3D('',#17669,#13983,#13984);
#12412=AXIS2_PLACEMENT_3D('',#17672,#13986,#13987);
#12413=AXIS2_PLACEMENT_3D('',#17673,#13988,#13989);
#12414=AXIS2_PLACEMENT_3D('',#17675,#13990,#13991);
#12415=AXIS2_PLACEMENT_3D('',#17678,#13993,#13994);
#12416=AXIS2_PLACEMENT_3D('',#17679,#13995,#13996);
#12417=AXIS2_PLACEMENT_3D('',#17681,#13998,#13999);
#12418=AXIS2_PLACEMENT_3D('',#17683,#14000,#14001);
#12419=AXIS2_PLACEMENT_3D('',#17686,#14003,#14004);
#12420=AXIS2_PLACEMENT_3D('',#17687,#14005,#14006);
#12421=AXIS2_PLACEMENT_3D('',#17691,#14008,#14009);
#12422=AXIS2_PLACEMENT_3D('',#17693,#14011,#14012);
#12423=AXIS2_PLACEMENT_3D('',#17695,#14013,#14014);
#12424=AXIS2_PLACEMENT_3D('',#17698,#14016,#14017);
#12425=AXIS2_PLACEMENT_3D('',#17699,#14018,#14019);
#12426=AXIS2_PLACEMENT_3D('',#17708,#14023,#14024);
#12427=AXIS2_PLACEMENT_3D('',#17710,#14026,#14027);
#12428=AXIS2_PLACEMENT_3D('',#17719,#14032,#14033);
#12429=AXIS2_PLACEMENT_3D('',#17727,#14038,#14039);
#12430=AXIS2_PLACEMENT_3D('',#17737,#14044,#14045);
#12431=AXIS2_PLACEMENT_3D('',#17738,#14046,#14047);
#12432=AXIS2_PLACEMENT_3D('',#17747,#14052,#14053);
#12433=AXIS2_PLACEMENT_3D('',#17756,#14057,#14058);
#12434=AXIS2_PLACEMENT_3D('',#17758,#14060,#14061);
#12435=AXIS2_PLACEMENT_3D('',#17761,#14062,#14063);
#12436=AXIS2_PLACEMENT_3D('',#17764,#14065,#14066);
#12437=AXIS2_PLACEMENT_3D('',#17765,#14067,#14068);
#12438=AXIS2_PLACEMENT_3D('',#17767,#14069,#14070);
#12439=AXIS2_PLACEMENT_3D('',#17771,#14072,#14073);
#12440=AXIS2_PLACEMENT_3D('',#17778,#14074,#14075);
#12441=AXIS2_PLACEMENT_3D('',#17787,#14079,#14080);
#12442=AXIS2_PLACEMENT_3D('',#17790,#14082,#14083);
#12443=AXIS2_PLACEMENT_3D('',#17791,#14084,#14085);
#12444=AXIS2_PLACEMENT_3D('',#17800,#14090,#14091);
#12445=AXIS2_PLACEMENT_3D('',#17811,#14098,#14099);
#12446=AXIS2_PLACEMENT_3D('',#17813,#14100,#14101);
#12447=AXIS2_PLACEMENT_3D('',#17816,#14103,#14104);
#12448=AXIS2_PLACEMENT_3D('',#17817,#14105,#14106);
#12449=AXIS2_PLACEMENT_3D('',#17821,#14108,#14109);
#12450=AXIS2_PLACEMENT_3D('',#17822,#14110,#14111);
#12451=AXIS2_PLACEMENT_3D('',#17823,#14112,#14113);
#12452=AXIS2_PLACEMENT_3D('',#17829,#14117,#14118);
#12453=AXIS2_PLACEMENT_3D('',#17835,#14122,#14123);
#12454=AXIS2_PLACEMENT_3D('',#17839,#14126,#14127);
#12455=AXIS2_PLACEMENT_3D('',#17840,#14128,#14129);
#12456=AXIS2_PLACEMENT_3D('',#17844,#14132,#14133);
#12457=AXIS2_PLACEMENT_3D('',#17845,#14134,#14135);
#12458=AXIS2_PLACEMENT_3D('',#17847,#14136,#14137);
#12459=AXIS2_PLACEMENT_3D('',#17850,#14139,#14140);
#12460=AXIS2_PLACEMENT_3D('',#17852,#14141,#14142);
#12461=AXIS2_PLACEMENT_3D('',#17856,#14144,#14145);
#12462=AXIS2_PLACEMENT_3D('',#17864,#14150,#14151);
#12463=AXIS2_PLACEMENT_3D('',#17867,#14153,#14154);
#12464=AXIS2_PLACEMENT_3D('',#17871,#14156,#14157);
#12465=AXIS2_PLACEMENT_3D('',#17873,#14159,#14160);
#12466=AXIS2_PLACEMENT_3D('',#17874,#14161,#14162);
#12467=AXIS2_PLACEMENT_3D('',#17879,#14164,#14165);
#12468=AXIS2_PLACEMENT_3D('',#17882,#14167,#14168);
#12469=AXIS2_PLACEMENT_3D('',#17884,#14169,#14170);
#12470=AXIS2_PLACEMENT_3D('',#17888,#14172,#14173);
#12471=AXIS2_PLACEMENT_3D('',#17892,#14175,#14176);
#12472=AXIS2_PLACEMENT_3D('',#17896,#14178,#14179);
#12473=AXIS2_PLACEMENT_3D('',#17897,#14180,#14181);
#12474=AXIS2_PLACEMENT_3D('',#17899,#14182,#14183);
#12475=AXIS2_PLACEMENT_3D('',#17903,#14185,#14186);
#12476=AXIS2_PLACEMENT_3D('',#17906,#14188,#14189);
#12477=AXIS2_PLACEMENT_3D('',#17907,#14190,#14191);
#12478=AXIS2_PLACEMENT_3D('',#17913,#14195,#14196);
#12479=AXIS2_PLACEMENT_3D('',#17922,#14201,#14202);
#12480=AXIS2_PLACEMENT_3D('',#17924,#14203,#14204);
#12481=AXIS2_PLACEMENT_3D('',#17927,#14206,#14207);
#12482=AXIS2_PLACEMENT_3D('',#17928,#14208,#14209);
#12483=AXIS2_PLACEMENT_3D('',#17930,#14210,#14211);
#12484=AXIS2_PLACEMENT_3D('',#17934,#14213,#14214);
#12485=AXIS2_PLACEMENT_3D('',#17938,#14216,#14217);
#12486=AXIS2_PLACEMENT_3D('',#17942,#14219,#14220);
#12487=AXIS2_PLACEMENT_3D('',#17946,#14222,#14223);
#12488=AXIS2_PLACEMENT_3D('',#17951,#14226,#14227);
#12489=AXIS2_PLACEMENT_3D('',#17953,#14228,#14229);
#12490=AXIS2_PLACEMENT_3D('',#17956,#14231,#14232);
#12491=AXIS2_PLACEMENT_3D('',#17960,#14234,#14235);
#12492=AXIS2_PLACEMENT_3D('',#17964,#14237,#14238);
#12493=AXIS2_PLACEMENT_3D('',#17967,#14241,#14242);
#12494=AXIS2_PLACEMENT_3D('',#17970,#14245,#14246);
#12495=AXIS2_PLACEMENT_3D('',#17973,#14249,#14250);
#12496=AXIS2_PLACEMENT_3D('',#17976,#14253,#14254);
#12497=AXIS2_PLACEMENT_3D('',#17979,#14257,#14258);
#12498=AXIS2_PLACEMENT_3D('',#17980,#14259,#14260);
#12499=AXIS2_PLACEMENT_3D('',#17985,#14263,#14264);
#12500=AXIS2_PLACEMENT_3D('',#17987,#14266,#14267);
#12501=AXIS2_PLACEMENT_3D('',#17991,#14269,#14270);
#12502=AXIS2_PLACEMENT_3D('',#17992,#14271,#14272);
#12503=AXIS2_PLACEMENT_3D('',#17993,#14273,#14274);
#12504=AXIS2_PLACEMENT_3D('',#17998,#14277,#14278);
#12505=AXIS2_PLACEMENT_3D('',#18001,#14280,#14281);
#12506=AXIS2_PLACEMENT_3D('',#18002,#14282,#14283);
#12507=AXIS2_PLACEMENT_3D('',#18005,#14284,#14285);
#12508=AXIS2_PLACEMENT_3D('',#18008,#14288,#14289);
#12509=AXIS2_PLACEMENT_3D('',#18014,#14293,#14294);
#12510=AXIS2_PLACEMENT_3D('',#18017,#14296,#14297);
#12511=AXIS2_PLACEMENT_3D('',#18018,#14298,#14299);
#12512=AXIS2_PLACEMENT_3D('',#18022,#14301,#14302);
#12513=AXIS2_PLACEMENT_3D('',#18024,#14304,#14305);
#12514=AXIS2_PLACEMENT_3D('',#18029,#14307,#14308);
#12515=AXIS2_PLACEMENT_3D('',#18033,#14311,#14312);
#12516=AXIS2_PLACEMENT_3D('',#18034,#14313,#14314);
#12517=AXIS2_PLACEMENT_3D('',#18040,#14318,#14319);
#12518=AXIS2_PLACEMENT_3D('',#18042,#14320,#14321);
#12519=AXIS2_PLACEMENT_3D('',#18044,#14323,#14324);
#12520=AXIS2_PLACEMENT_3D('',#18045,#14325,#14326);
#12521=AXIS2_PLACEMENT_3D('',#18049,#14329,#14330);
#12522=AXIS2_PLACEMENT_3D('',#18058,#14335,#14336);
#12523=AXIS2_PLACEMENT_3D('',#18062,#14338,#14339);
#12524=AXIS2_PLACEMENT_3D('',#18069,#14340,#14341);
#12525=AXIS2_PLACEMENT_3D('',#18070,#14342,#14343);
#12526=AXIS2_PLACEMENT_3D('',#18071,#14344,#14345);
#12527=AXIS2_PLACEMENT_3D('',#18072,#14346,#14347);
#12528=AXIS2_PLACEMENT_3D('',#18073,#14348,#14349);
#12529=AXIS2_PLACEMENT_3D('',#18074,#14350,#14351);
#12530=AXIS2_PLACEMENT_3D('',#18083,#14356,#14357);
#12531=AXIS2_PLACEMENT_3D('',#18091,#14361,#14362);
#12532=AXIS2_PLACEMENT_3D('',#18092,#14363,#14364);
#12533=AXIS2_PLACEMENT_3D('',#18093,#14365,#14366);
#12534=AXIS2_PLACEMENT_3D('',#18096,#14368,#14369);
#12535=AXIS2_PLACEMENT_3D('',#18098,#14371,#14372);
#12536=AXIS2_PLACEMENT_3D('',#18105,#14375,#14376);
#12537=AXIS2_PLACEMENT_3D('',#18107,#14378,#14379);
#12538=AXIS2_PLACEMENT_3D('',#18111,#14382,#14383);
#12539=AXIS2_PLACEMENT_3D('',#18112,#14384,#14385);
#12540=AXIS2_PLACEMENT_3D('',#18113,#14386,#14387);
#12541=AXIS2_PLACEMENT_3D('',#18117,#14390,#14391);
#12542=AXIS2_PLACEMENT_3D('',#18118,#14392,#14393);
#12543=AXIS2_PLACEMENT_3D('',#18119,#14394,#14395);
#12544=AXIS2_PLACEMENT_3D('',#18120,#14396,#14397);
#12545=AXIS2_PLACEMENT_3D('',#18121,#14398,#14399);
#12546=AXIS2_PLACEMENT_3D('',#18122,#14400,#14401);
#12547=AXIS2_PLACEMENT_3D('',#18128,#14405,#14406);
#12548=AXIS2_PLACEMENT_3D('',#18132,#14409,#14410);
#12549=AXIS2_PLACEMENT_3D('',#18136,#14413,#14414);
#12550=AXIS2_PLACEMENT_3D('',#18142,#14418,#14419);
#12551=AXIS2_PLACEMENT_3D('',#18144,#14420,#14421);
#12552=AXIS2_PLACEMENT_3D('',#18147,#14423,#14424);
#12553=AXIS2_PLACEMENT_3D('',#18148,#14425,#14426);
#12554=AXIS2_PLACEMENT_3D('',#18149,#14427,#14428);
#12555=AXIS2_PLACEMENT_3D('',#18151,#14429,#14430);
#12556=AXIS2_PLACEMENT_3D('',#18153,#14432,#14433);
#12557=AXIS2_PLACEMENT_3D('',#18154,#14434,#14435);
#12558=AXIS2_PLACEMENT_3D('',#18155,#14436,#14437);
#12559=AXIS2_PLACEMENT_3D('',#18156,#14438,#14439);
#12560=AXIS2_PLACEMENT_3D('',#18159,#14442,#14443);
#12561=AXIS2_PLACEMENT_3D('',#18166,#14447,#14448);
#12562=AXIS2_PLACEMENT_3D('',#18167,#14449,#14450);
#12563=AXIS2_PLACEMENT_3D('',#18168,#14451,#14452);
#12564=AXIS2_PLACEMENT_3D('',#18172,#14455,#14456);
#12565=AXIS2_PLACEMENT_3D('',#18173,#14457,#14458);
#12566=AXIS2_PLACEMENT_3D('',#18175,#14460,#14461);
#12567=AXIS2_PLACEMENT_3D('',#18178,#14464,#14465);
#12568=AXIS2_PLACEMENT_3D('',#18179,#14466,#14467);
#12569=AXIS2_PLACEMENT_3D('',#18180,#14468,#14469);
#12570=AXIS2_PLACEMENT_3D('',#18181,#14470,#14471);
#12571=AXIS2_PLACEMENT_3D('',#18182,#14472,#14473);
#12572=AXIS2_PLACEMENT_3D('',#18185,#14474,#14475);
#12573=AXIS2_PLACEMENT_3D('',#18191,#14479,#14480);
#12574=AXIS2_PLACEMENT_3D('',#18195,#14483,#14484);
#12575=AXIS2_PLACEMENT_3D('',#18196,#14485,#14486);
#12576=AXIS2_PLACEMENT_3D('',#18197,#14487,#14488);
#12577=AXIS2_PLACEMENT_3D('',#18203,#14492,#14493);
#12578=AXIS2_PLACEMENT_3D('',#18207,#14496,#14497);
#12579=AXIS2_PLACEMENT_3D('',#18208,#14498,#14499);
#12580=AXIS2_PLACEMENT_3D('',#18210,#14501,#14502);
#12581=AXIS2_PLACEMENT_3D('',#18211,#14503,#14504);
#12582=AXIS2_PLACEMENT_3D('',#18212,#14505,#14506);
#12583=AXIS2_PLACEMENT_3D('',#18213,#14507,#14508);
#12584=AXIS2_PLACEMENT_3D('',#18214,#14509,#14510);
#12585=AXIS2_PLACEMENT_3D('',#18215,#14511,#14512);
#12586=AXIS2_PLACEMENT_3D('',#18216,#14513,#14514);
#12587=AXIS2_PLACEMENT_3D('',#18217,#14515,#14516);
#12588=AXIS2_PLACEMENT_3D('',#18218,#14517,#14518);
#12589=AXIS2_PLACEMENT_3D('',#18227,#14523,#14524);
#12590=AXIS2_PLACEMENT_3D('',#18228,#14525,#14526);
#12591=AXIS2_PLACEMENT_3D('',#18229,#14527,#14528);
#12592=AXIS2_PLACEMENT_3D('',#18238,#14533,#14534);
#12593=AXIS2_PLACEMENT_3D('',#18240,#14535,#14536);
#12594=AXIS2_PLACEMENT_3D('',#18243,#14538,#14539);
#12595=AXIS2_PLACEMENT_3D('',#18245,#14540,#14541);
#12596=AXIS2_PLACEMENT_3D('',#18248,#14543,#14544);
#12597=AXIS2_PLACEMENT_3D('',#18249,#14545,#14546);
#12598=AXIS2_PLACEMENT_3D('',#18253,#14548,#14549);
#12599=AXIS2_PLACEMENT_3D('',#18255,#14550,#14551);
#12600=AXIS2_PLACEMENT_3D('',#18258,#14553,#14554);
#12601=AXIS2_PLACEMENT_3D('',#18259,#14555,#14556);
#12602=AXIS2_PLACEMENT_3D('',#18260,#14557,#14558);
#12603=AXIS2_PLACEMENT_3D('',#18261,#14559,#14560);
#12604=AXIS2_PLACEMENT_3D('',#18262,#14561,#14562);
#12605=AXIS2_PLACEMENT_3D('',#18263,#14563,#14564);
#12606=AXIS2_PLACEMENT_3D('',#18264,#14565,#14566);
#12607=AXIS2_PLACEMENT_3D('',#18265,#14567,#14568);
#12608=AXIS2_PLACEMENT_3D('',#18266,#14569,#14570);
#12609=AXIS2_PLACEMENT_3D('',#18267,#14571,#14572);
#12610=AXIS2_PLACEMENT_3D('',#18268,#14573,#14574);
#12611=AXIS2_PLACEMENT_3D('',#18269,#14575,#14576);
#12612=AXIS2_PLACEMENT_3D('',#18270,#14577,#14578);
#12613=AXIS2_PLACEMENT_3D('',#18271,#14579,#14580);
#12614=AXIS2_PLACEMENT_3D('',#18272,#14581,#14582);
#12615=AXIS2_PLACEMENT_3D('',#18273,#14583,#14584);
#12616=AXIS2_PLACEMENT_3D('',#18274,#14585,#14586);
#12617=AXIS2_PLACEMENT_3D('',#18275,#14587,#14588);
#12618=AXIS2_PLACEMENT_3D('',#18276,#14589,#14590);
#12619=AXIS2_PLACEMENT_3D('',#18277,#14591,#14592);
#12620=AXIS2_PLACEMENT_3D('',#18278,#14593,#14594);
#12621=AXIS2_PLACEMENT_3D('',#18279,#14595,#14596);
#12622=AXIS2_PLACEMENT_3D('',#18280,#14597,#14598);
#12623=AXIS2_PLACEMENT_3D('',#18281,#14599,#14600);
#12624=AXIS2_PLACEMENT_3D('',#18282,#14601,#14602);
#12625=AXIS2_PLACEMENT_3D('',#18283,#14603,#14604);
#12626=AXIS2_PLACEMENT_3D('',#18284,#14605,#14606);
#12627=AXIS2_PLACEMENT_3D('',#18295,#14607,#14608);
#12628=AXIS2_PLACEMENT_3D('',#18318,#14609,#14610);
#12629=AXIS2_PLACEMENT_3D('',#18335,#14611,#14612);
#12630=AXIS2_PLACEMENT_3D('',#18352,#14613,#14614);
#12631=AXIS2_PLACEMENT_3D('',#18353,#14615,#14616);
#12632=AXIS2_PLACEMENT_3D('',#18354,#14617,#14618);
#12633=AXIS2_PLACEMENT_3D('',#18355,#14619,#14620);
#12634=AXIS2_PLACEMENT_3D('',#18356,#14621,#14622);
#12635=AXIS2_PLACEMENT_3D('',#18357,#14623,#14624);
#12636=AXIS2_PLACEMENT_3D('',#18430,#14625,#14626);
#12637=AXIS2_PLACEMENT_3D('',#18431,#14627,#14628);
#12638=AXIS2_PLACEMENT_3D('',#18432,#14629,#14630);
#12639=AXIS2_PLACEMENT_3D('',#18433,#14631,#14632);
#12640=AXIS2_PLACEMENT_3D('',#18434,#14633,#14634);
#12641=AXIS2_PLACEMENT_3D('',#18435,#14635,#14636);
#12642=AXIS2_PLACEMENT_3D('',#18436,#14637,#14638);
#12643=AXIS2_PLACEMENT_3D('',#18437,#14639,#14640);
#12644=AXIS2_PLACEMENT_3D('',#18444,#14641,#14642);
#12645=AXIS2_PLACEMENT_3D('',#18451,#14643,#14644);
#12646=AXIS2_PLACEMENT_3D('',#18458,#14645,#14646);
#12647=AXIS2_PLACEMENT_3D('',#18465,#14647,#14648);
#12648=AXIS2_PLACEMENT_3D('',#18466,#14649,#14650);
#12649=AXIS2_PLACEMENT_3D('',#18467,#14651,#14652);
#12650=AXIS2_PLACEMENT_3D('',#18468,#14653,#14654);
#12651=AXIS2_PLACEMENT_3D('',#18469,#14655,#14656);
#13734=DIRECTION('axis',(0.,0.,1.));
#13735=DIRECTION('refdir',(1.,0.,0.));
#13736=DIRECTION('center_axis',(0.,0.,-1.));
#13737=DIRECTION('ref_axis',(-1.,0.,0.));
#13738=DIRECTION('center_axis',(0.,0.,-1.));
#13739=DIRECTION('ref_axis',(1.,0.,0.));
#13740=DIRECTION('',(-0.707106781186543,8.65956056235488E-17,0.707106781186552));
#13741=DIRECTION('center_axis',(0.,0.,1.));
#13742=DIRECTION('ref_axis',(1.,0.,0.));
#13743=DIRECTION('center_axis',(0.,0.,1.));
#13744=DIRECTION('ref_axis',(1.,0.,0.));
#13745=DIRECTION('center_axis',(0.,0.,1.));
#13746=DIRECTION('ref_axis',(-1.,0.,0.));
#13747=DIRECTION('',(0.707106781186543,8.65956056235488E-17,-0.707106781186552));
#13748=DIRECTION('center_axis',(0.,0.,-1.));
#13749=DIRECTION('ref_axis',(-1.,0.,0.));
#13750=DIRECTION('center_axis',(0.,0.,-1.));
#13751=DIRECTION('ref_axis',(-1.,0.,0.));
#13752=DIRECTION('center_axis',(0.,0.,-1.));
#13753=DIRECTION('ref_axis',(1.,0.,0.));
#13754=DIRECTION('',(-0.707106781186552,8.65956056235498E-17,0.707106781186544));
#13755=DIRECTION('center_axis',(0.,0.,1.));
#13756=DIRECTION('ref_axis',(1.,0.,0.));
#13757=DIRECTION('center_axis',(0.,0.,-1.));
#13758=DIRECTION('ref_axis',(-1.,0.,0.));
#13759=DIRECTION('center_axis',(0.,0.,-1.));
#13760=DIRECTION('ref_axis',(1.,0.,0.));
#13761=DIRECTION('',(-0.70710678118656,8.65956056235508E-17,0.707106781186535));
#13762=DIRECTION('center_axis',(0.,0.,1.));
#13763=DIRECTION('ref_axis',(1.,0.,0.));
#13764=DIRECTION('center_axis',(0.,0.,1.));
#13765=DIRECTION('ref_axis',(1.,0.,0.));
#13766=DIRECTION('center_axis',(0.,0.,1.));
#13767=DIRECTION('ref_axis',(-1.,0.,0.));
#13768=DIRECTION('',(0.707106781186543,8.65956056235488E-17,-0.707106781186552));
#13769=DIRECTION('center_axis',(0.,0.,-1.));
#13770=DIRECTION('ref_axis',(-1.,0.,0.));
#13771=DIRECTION('center_axis',(0.,0.,1.));
#13772=DIRECTION('ref_axis',(1.,0.,0.));
#13773=DIRECTION('center_axis',(0.,0.,1.));
#13774=DIRECTION('ref_axis',(-1.,0.,0.));
#13775=DIRECTION('',(0.70710678118658,8.65956056235533E-17,-0.707106781186515));
#13776=DIRECTION('center_axis',(0.,0.,-1.));
#13777=DIRECTION('ref_axis',(-1.,0.,0.));
#13778=DIRECTION('center_axis',(-1.26920068081332E-33,-4.21788745889624E-34,
1.));
#13779=DIRECTION('ref_axis',(1.,-5.35334563442508E-67,1.26920068081332E-33));
#13780=DIRECTION('center_axis',(0.,0.,1.));
#13781=DIRECTION('ref_axis',(-1.,4.00913870003528E-14,0.));
#13782=DIRECTION('',(1.26920068081332E-33,4.21788745889624E-34,-1.));
#13783=DIRECTION('center_axis',(0.,0.,-1.));
#13784=DIRECTION('ref_axis',(-1.,0.,0.));
#13785=DIRECTION('',(8.7532076796714E-18,-2.63391976542839E-17,-1.));
#13786=DIRECTION('center_axis',(0.,-1.,0.));
#13787=DIRECTION('ref_axis',(0.,0.,-1.));
#13788=DIRECTION('center_axis',(0.,1.,0.));
#13789=DIRECTION('ref_axis',(0.,0.,-1.));
#13790=DIRECTION('center_axis',(0.12947657529132,-2.29349521067294E-15,
0.991582480911614));
#13791=DIRECTION('ref_axis',(0.991582480911614,5.32481111024183E-30,-0.12947657529132));
#13792=DIRECTION('center_axis',(0.,-1.,0.));
#13793=DIRECTION('ref_axis',(0.,0.,-1.));
#13794=DIRECTION('center_axis',(-2.31296463463574E-15,0.,-1.));
#13795=DIRECTION('ref_axis',(-1.,0.,2.31296463463574E-15));
#13796=DIRECTION('center_axis',(0.,0.,1.));
#13797=DIRECTION('ref_axis',(1.,0.,0.));
#13798=DIRECTION('center_axis',(0.,0.,1.));
#13799=DIRECTION('ref_axis',(1.,0.,0.));
#13800=DIRECTION('center_axis',(0.,1.,0.));
#13801=DIRECTION('ref_axis',(-1.,0.,0.));
#13802=DIRECTION('center_axis',(0.,0.,-1.));
#13803=DIRECTION('ref_axis',(1.,0.,0.));
#13804=DIRECTION('center_axis',(0.,0.,1.));
#13805=DIRECTION('ref_axis',(1.,0.,0.));
#13806=DIRECTION('center_axis',(0.,0.,1.));
#13807=DIRECTION('ref_axis',(1.,0.,0.));
#13808=DIRECTION('center_axis',(0.,1.,0.));
#13809=DIRECTION('ref_axis',(-1.,0.,0.));
#13810=DIRECTION('center_axis',(0.,0.,-1.));
#13811=DIRECTION('ref_axis',(1.,0.,0.));
#13812=DIRECTION('center_axis',(0.,0.,-1.));
#13813=DIRECTION('ref_axis',(-1.,0.,0.));
#13814=DIRECTION('center_axis',(0.,0.,-1.));
#13815=DIRECTION('ref_axis',(-1.,0.,0.));
#13816=DIRECTION('center_axis',(0.,1.,0.));
#13817=DIRECTION('ref_axis',(1.,0.,0.));
#13818=DIRECTION('center_axis',(0.,0.,1.));
#13819=DIRECTION('ref_axis',(-1.,0.,0.));
#13820=DIRECTION('center_axis',(0.,0.,-1.));
#13821=DIRECTION('ref_axis',(-1.,0.,0.));
#13822=DIRECTION('center_axis',(0.,0.,-1.));
#13823=DIRECTION('ref_axis',(-1.,0.,0.));
#13824=DIRECTION('center_axis',(0.,1.,0.));
#13825=DIRECTION('ref_axis',(1.,0.,0.));
#13826=DIRECTION('center_axis',(0.,0.,1.));
#13827=DIRECTION('ref_axis',(-1.,0.,0.));
#13828=DIRECTION('center_axis',(0.,0.,-1.));
#13829=DIRECTION('ref_axis',(-0.00404500334087533,-0.999991818940521,0.));
#13830=DIRECTION('center_axis',(0.,0.,-1.));
#13831=DIRECTION('ref_axis',(-1.,0.,0.));
#13832=DIRECTION('center_axis',(0.960335432337036,-0.27884737294448,-7.73956934497999E-15));
#13833=DIRECTION('ref_axis',(0.27884737294448,0.960335432337036,3.94430452610506E-31));
#13834=DIRECTION('center_axis',(0.,0.,1.));
#13835=DIRECTION('ref_axis',(-1.,0.,0.));
#13836=DIRECTION('center_axis',(0.,0.,1.));
#13837=DIRECTION('ref_axis',(-1.,0.,0.));
#13838=DIRECTION('center_axis',(-0.962559864875271,-0.271069191409314,0.));
#13839=DIRECTION('ref_axis',(0.271069191409314,-0.962559864875271,0.));
#13840=DIRECTION('center_axis',(0.,0.,1.));
#13841=DIRECTION('ref_axis',(-0.00404500334087533,-0.999991818940521,0.));
#13842=DIRECTION('center_axis',(0.,0.,1.));
#13843=DIRECTION('ref_axis',(1.,0.,0.));
#13844=DIRECTION('center_axis',(-0.96255986487527,-0.271069191409318,3.76184071961435E-15));
#13845=DIRECTION('ref_axis',(0.271069191409318,-0.96255986487527,0.));
#13846=DIRECTION('center_axis',(0.,0.,-1.));
#13847=DIRECTION('ref_axis',(1.,0.,0.));
#13848=DIRECTION('center_axis',(0.,0.,-1.));
#13849=DIRECTION('ref_axis',(1.,0.,0.));
#13850=DIRECTION('center_axis',(0.960335432337038,-0.278847372944473,0.));
#13851=DIRECTION('ref_axis',(0.278847372944473,0.960335432337038,0.));
#13852=DIRECTION('center_axis',(0.,0.,1.));
#13853=DIRECTION('ref_axis',(1.,0.,0.));
#13854=DIRECTION('center_axis',(0.,0.,1.));
#13855=DIRECTION('ref_axis',(1.,0.,0.));
#13856=DIRECTION('center_axis',(0.,1.,0.));
#13857=DIRECTION('ref_axis',(-1.,0.,0.));
#13858=DIRECTION('center_axis',(0.,0.,-1.));
#13859=DIRECTION('ref_axis',(1.,0.,0.));
#13860=DIRECTION('center_axis',(0.,0.,-1.));
#13861=DIRECTION('ref_axis',(1.,0.,0.));
#13862=DIRECTION('center_axis',(0.,0.,-1.));
#13863=DIRECTION('ref_axis',(-1.,0.,0.));
#13864=DIRECTION('center_axis',(0.,0.,-1.));
#13865=DIRECTION('ref_axis',(-1.,0.,0.));
#13866=DIRECTION('center_axis',(0.,1.,0.));
#13867=DIRECTION('ref_axis',(1.,0.,0.));
#13868=DIRECTION('center_axis',(0.,0.,1.));
#13869=DIRECTION('ref_axis',(-1.,0.,0.));
#13870=DIRECTION('center_axis',(0.,0.,1.));
#13871=DIRECTION('ref_axis',(1.,0.,0.));
#13872=DIRECTION('center_axis',(0.,0.,1.));
#13873=DIRECTION('ref_axis',(1.,0.,0.));
#13874=DIRECTION('center_axis',(0.,0.,1.));
#13875=DIRECTION('ref_axis',(1.,0.,0.));
#13876=DIRECTION('center_axis',(0.,1.,0.));
#13877=DIRECTION('ref_axis',(-1.,0.,0.));
#13878=DIRECTION('center_axis',(0.,0.,-1.));
#13879=DIRECTION('ref_axis',(1.,0.,0.));
#13880=DIRECTION('center_axis',(0.,0.,-1.));
#13881=DIRECTION('ref_axis',(-1.,0.,0.));
#13882=DIRECTION('center_axis',(0.,0.,-1.));
#13883=DIRECTION('ref_axis',(-1.,0.,0.));
#13884=DIRECTION('center_axis',(0.,0.,-1.));
#13885=DIRECTION('ref_axis',(-1.,0.,0.));
#13886=DIRECTION('center_axis',(0.,1.,0.));
#13887=DIRECTION('ref_axis',(1.,0.,0.));
#13888=DIRECTION('center_axis',(0.,0.,1.));
#13889=DIRECTION('ref_axis',(-1.,0.,0.));
#13890=DIRECTION('center_axis',(0.,1.,0.));
#13891=DIRECTION('ref_axis',(0.,0.,1.));
#13892=DIRECTION('center_axis',(0.,1.,3.85494105772624E-16));
#13893=DIRECTION('ref_axis',(0.,-3.85494105772624E-16,1.));
#13894=DIRECTION('',(0.,-1.,0.));
#13895=DIRECTION('center_axis',(0.,-1.,0.));
#13896=DIRECTION('ref_axis',(0.,0.,-1.));
#13897=DIRECTION('center_axis',(-0.0915537643933219,0.707106781186538,-0.70115469635839));
#13898=DIRECTION('ref_axis',(0.091553764391814,0.707106781186557,0.701154696358567));
#13899=DIRECTION('',(0.,1.,0.));
#13900=DIRECTION('center_axis',(0.,1.,0.));
#13901=DIRECTION('ref_axis',(0.,0.,-1.));
#13902=DIRECTION('center_axis',(0.,-1.,0.));
#13903=DIRECTION('ref_axis',(0.,0.,-1.));
#13904=DIRECTION('center_axis',(0.,-1.,0.));
#13905=DIRECTION('ref_axis',(0.,0.,-1.));
#13906=DIRECTION('center_axis',(0.,0.,1.));
#13907=DIRECTION('ref_axis',(1.,0.,0.));
#13908=DIRECTION('center_axis',(0.,1.,0.));
#13909=DIRECTION('ref_axis',(1.02798428206033E-15,0.,-1.));
#13910=DIRECTION('center_axis',(-0.129476575291326,0.,-0.991582480911613));
#13911=DIRECTION('ref_axis',(-0.991582480911613,0.,0.129476575291326));
#13912=DIRECTION('center_axis',(0.,0.,1.));
#13913=DIRECTION('ref_axis',(1.,0.,0.));
#13914=DIRECTION('center_axis',(0.,0.,-1.));
#13915=DIRECTION('ref_axis',(-1.,0.,0.));
#13916=DIRECTION('',(0.,0.,1.));
#13917=DIRECTION('center_axis',(0.,0.,1.));
#13918=DIRECTION('ref_axis',(1.,0.,0.));
#13919=DIRECTION('center_axis',(0.,0.,-1.));
#13920=DIRECTION('ref_axis',(-1.,0.,0.));
#13921=DIRECTION('',(0.,0.,1.));
#13922=DIRECTION('center_axis',(0.,0.,-1.));
#13923=DIRECTION('ref_axis',(-1.,0.,0.));
#13924=DIRECTION('',(0.,0.,1.));
#13925=DIRECTION('center_axis',(0.,0.,-1.));
#13926=DIRECTION('ref_axis',(-1.,0.,0.));
#13927=DIRECTION('',(0.,0.,1.));
#13928=DIRECTION('center_axis',(0.,-1.,0.));
#13929=DIRECTION('ref_axis',(0.,0.,-1.));
#13930=DIRECTION('',(0.,-1.,0.));
#13931=DIRECTION('center_axis',(-8.08177633281312E-16,0.958646866278096,
0.284598288426311));
#13932=DIRECTION('ref_axis',(1.40325551131645E-13,-0.284598288426311,0.958646866278096));
#13933=DIRECTION('',(0.,-1.,0.));
#13934=DIRECTION('center_axis',(0.,0.,1.));
#13935=DIRECTION('ref_axis',(1.,0.,0.));
#13936=DIRECTION('',(0.,0.,-1.));
#13937=DIRECTION('center_axis',(0.,0.,1.));
#13938=DIRECTION('ref_axis',(1.,0.,0.));
#13939=DIRECTION('center_axis',(0.,0.,1.));
#13940=DIRECTION('ref_axis',(1.,0.,0.));
#13941=DIRECTION('center_axis',(0.,0.,1.));
#13942=DIRECTION('ref_axis',(1.,0.,0.));
#13943=DIRECTION('',(0.,0.,1.));
#13944=DIRECTION('center_axis',(0.,0.,-1.));
#13945=DIRECTION('ref_axis',(-1.,0.,0.));
#13946=DIRECTION('center_axis',(0.,0.,1.));
#13947=DIRECTION('ref_axis',(1.,0.,0.));
#13948=DIRECTION('center_axis',(0.,0.,1.));
#13949=DIRECTION('ref_axis',(1.,0.,0.));
#13950=DIRECTION('',(0.,0.,1.));
#13951=DIRECTION('center_axis',(0.,0.,-1.));
#13952=DIRECTION('ref_axis',(-1.,0.,0.));
#13953=DIRECTION('center_axis',(0.,0.,1.));
#13954=DIRECTION('ref_axis',(1.,0.,0.));
#13955=DIRECTION('center_axis',(0.,0.,1.));
#13956=DIRECTION('ref_axis',(1.,0.,0.));
#13957=DIRECTION('',(0.,0.,1.));
#13958=DIRECTION('center_axis',(0.,0.,-1.));
#13959=DIRECTION('ref_axis',(-1.,0.,0.));
#13960=DIRECTION('center_axis',(0.,0.,1.));
#13961=DIRECTION('ref_axis',(1.,0.,0.));
#13962=DIRECTION('',(0.,0.,-1.));
#13963=DIRECTION('center_axis',(0.,0.,1.));
#13964=DIRECTION('ref_axis',(1.,0.,0.));
#13965=DIRECTION('',(0.,0.,-1.));
#13966=DIRECTION('center_axis',(0.,0.,1.));
#13967=DIRECTION('ref_axis',(1.,0.,0.));
#13968=DIRECTION('',(0.,0.,-1.));
#13969=DIRECTION('center_axis',(0.,0.,-1.));
#13970=DIRECTION('ref_axis',(-1.,0.,0.));
#13971=DIRECTION('',(0.,0.,1.));
#13972=DIRECTION('center_axis',(0.,0.,1.));
#13973=DIRECTION('ref_axis',(1.,0.,0.));
#13974=DIRECTION('center_axis',(0.,0.,-1.));
#13975=DIRECTION('ref_axis',(-1.,0.,0.));
#13976=DIRECTION('center_axis',(0.,0.,1.));
#13977=DIRECTION('ref_axis',(1.,0.,0.));
#13978=DIRECTION('',(0.,0.,-1.));
#13979=DIRECTION('center_axis',(0.,0.,-1.));
#13980=DIRECTION('ref_axis',(-1.,0.,0.));
#13981=DIRECTION('center_axis',(0.,0.,-1.));
#13982=DIRECTION('ref_axis',(-1.,0.,0.));
#13983=DIRECTION('center_axis',(0.,0.,1.));
#13984=DIRECTION('ref_axis',(1.,0.,0.));
#13985=DIRECTION('',(0.,0.,-1.));
#13986=DIRECTION('center_axis',(0.,0.,-1.));
#13987=DIRECTION('ref_axis',(-1.,0.,0.));
#13988=DIRECTION('center_axis',(0.,0.,-1.));
#13989=DIRECTION('ref_axis',(-1.,0.,0.));
#13990=DIRECTION('center_axis',(0.,0.,1.));
#13991=DIRECTION('ref_axis',(1.,0.,0.));
#13992=DIRECTION('',(0.,0.,-1.));
#13993=DIRECTION('center_axis',(0.,0.,-1.));
#13994=DIRECTION('ref_axis',(-1.,0.,0.));
#13995=DIRECTION('center_axis',(0.,0.,-1.));
#13996=DIRECTION('ref_axis',(-1.,0.,0.));
#13997=DIRECTION('',(0.,0.,1.));
#13998=DIRECTION('center_axis',(0.,-1.,0.));
#13999=DIRECTION('ref_axis',(0.,0.,-1.));
#14000=DIRECTION('center_axis',(0.,-1.,0.));
#14001=DIRECTION('ref_axis',(0.,0.,-1.));
#14002=DIRECTION('',(0.,-1.,0.));
#14003=DIRECTION('center_axis',(0.,1.,0.));
#14004=DIRECTION('ref_axis',(0.,0.,-1.));
#14005=DIRECTION('center_axis',(0.,-1.,0.));
#14006=DIRECTION('ref_axis',(0.,0.,-1.));
#14007=DIRECTION('',(0.,-1.,0.));
#14008=DIRECTION('center_axis',(-2.75380126257971E-15,0.958646866278097,
0.284598288426308));
#14009=DIRECTION('ref_axis',(1.36429802923528E-12,-0.284598288426308,0.958646866278097));
#14010=DIRECTION('',(0.,-1.,0.));
#14011=DIRECTION('center_axis',(0.,-1.,0.));
#14012=DIRECTION('ref_axis',(0.,0.,-1.));
#14013=DIRECTION('center_axis',(0.,1.,0.));
#14014=DIRECTION('ref_axis',(0.,0.,1.));
#14015=DIRECTION('',(0.,-1.,0.));
#14016=DIRECTION('center_axis',(0.,-1.,0.));
#14017=DIRECTION('ref_axis',(0.,0.,-1.));
#14018=DIRECTION('center_axis',(0.,-1.,0.));
#14019=DIRECTION('ref_axis',(0.,0.,-1.));
#14020=DIRECTION('',(2.52323414687536E-15,0.,1.));
#14021=DIRECTION('',(1.,0.,0.));
#14022=DIRECTION('',(0.,0.,1.));
#14023=DIRECTION('center_axis',(0.,1.,0.));
#14024=DIRECTION('ref_axis',(0.,0.,-1.));
#14025=DIRECTION('',(1.,0.,0.));
#14026=DIRECTION('center_axis',(0.,-1.,0.));
#14027=DIRECTION('ref_axis',(0.,0.,-1.));
#14028=DIRECTION('',(1.,0.,0.));
#14029=DIRECTION('',(0.,0.,1.));
#14030=DIRECTION('',(1.,0.,0.));
#14031=DIRECTION('',(0.,0.,-1.));
#14032=DIRECTION('center_axis',(0.,-1.,0.));
#14033=DIRECTION('ref_axis',(0.,0.,-1.));
#14034=DIRECTION('',(-0.129476575291326,0.,-0.991582480911613));
#14035=DIRECTION('',(1.,0.,0.));
#14036=DIRECTION('',(-0.129476575291322,0.,-0.991582480911614));
#14037=DIRECTION('',(1.,0.,0.));
#14038=DIRECTION('center_axis',(0.,1.,0.));
#14039=DIRECTION('ref_axis',(0.,0.,1.));
#14040=DIRECTION('',(0.,0.,-1.));
#14041=DIRECTION('',(-1.,0.,0.));
#14042=DIRECTION('',(2.52323414687536E-15,0.,-1.));
#14043=DIRECTION('',(1.,0.,0.));
#14044=DIRECTION('center_axis',(0.,1.,0.));
#14045=DIRECTION('ref_axis',(0.,0.,1.));
#14046=DIRECTION('center_axis',(0.,1.,0.));
#14047=DIRECTION('ref_axis',(0.,0.,1.));
#14048=DIRECTION('',(1.,0.,0.));
#14049=DIRECTION('',(0.,0.,1.));
#14050=DIRECTION('',(1.,0.,0.));
#14051=DIRECTION('',(0.,0.,-1.));
#14052=DIRECTION('center_axis',(0.,1.,0.));
#14053=DIRECTION('ref_axis',(0.,0.,1.));
#14054=DIRECTION('',(-0.129476575291322,0.,0.991582480911614));
#14055=DIRECTION('',(-1.,0.,0.));
#14056=DIRECTION('',(-0.129476575291321,0.,0.991582480911614));
#14057=DIRECTION('center_axis',(0.,1.,0.));
#14058=DIRECTION('ref_axis',(0.,0.,1.));
#14059=DIRECTION('',(1.,0.,0.));
#14060=DIRECTION('center_axis',(0.,0.,1.));
#14061=DIRECTION('ref_axis',(1.,0.,0.));
#14062=DIRECTION('center_axis',(-0.671022843491604,-0.222998528050286,0.707106781186441));
#14063=DIRECTION('ref_axis',(0.671022846456233,0.222998519128768,0.707106781186654));
#14064=DIRECTION('',(0.,0.,1.));
#14065=DIRECTION('center_axis',(0.,0.,1.));
#14066=DIRECTION('ref_axis',(-1.,0.,0.));
#14067=DIRECTION('center_axis',(0.,0.,1.));
#14068=DIRECTION('ref_axis',(-1.,3.91353616180368E-14,0.));
#14069=DIRECTION('center_axis',(0.,0.,1.));
#14070=DIRECTION('ref_axis',(-1.,-1.06858966120171E-14,0.));
#14071=DIRECTION('',(0.,0.,1.));
#14072=DIRECTION('center_axis',(0.,0.,-1.));
#14073=DIRECTION('ref_axis',(-1.,0.,0.));
#14074=DIRECTION('center_axis',(-0.315367542755717,0.948969605928568,-2.77555756156289E-17));
#14075=DIRECTION('ref_axis',(-0.948969605928567,-0.315367542755717,0.));
#14076=DIRECTION('',(0.671022843492016,0.222998528048706,0.707106781186547));
#14077=DIRECTION('',(-0.948969605928567,-0.315367542755717,0.));
#14078=DIRECTION('',(0.671022843492016,0.222998528048706,-0.707106781186548));
#14079=DIRECTION('center_axis',(0.315367542755717,-0.948969605928567,2.77555756156289E-17));
#14080=DIRECTION('ref_axis',(-0.948969605928567,-0.315367542755717,3.08148791101958E-33));
#14081=DIRECTION('',(0.948969605928567,0.315367542755717,5.68761795402233E-17));
#14082=DIRECTION('center_axis',(0.315367542755717,-0.948969605928567,2.77555756156289E-17));
#14083=DIRECTION('ref_axis',(-0.948969605928567,-0.315367542755718,1.57107031786579E-15));
#14084=DIRECTION('center_axis',(0.,-1.,0.));
#14085=DIRECTION('ref_axis',(0.,0.,-1.));
#14086=DIRECTION('',(1.,0.,0.));
#14087=DIRECTION('',(0.,0.,-1.));
#14088=DIRECTION('',(1.,0.,0.));
#14089=DIRECTION('',(0.,0.,1.));
#14090=DIRECTION('center_axis',(0.,-0.958646866278097,-0.28459828842631));
#14091=DIRECTION('ref_axis',(0.,0.28459828842631,-0.958646866278097));
#14092=DIRECTION('',(0.,-0.28459828842631,0.958646866278097));
#14093=DIRECTION('',(1.,0.,0.));
#14094=DIRECTION('',(2.41889050778795E-15,-0.28459828842631,0.958646866278097));
#14095=DIRECTION('',(-0.124206667879909,0.28239446456039,-0.95122345957184));
#14096=DIRECTION('',(1.,0.,0.));
#14097=DIRECTION('',(-0.124206667879913,0.28239446456039,-0.95122345957184));
#14098=DIRECTION('center_axis',(1.,0.,0.));
#14099=DIRECTION('ref_axis',(0.,0.,-1.));
#14100=DIRECTION('center_axis',(1.,0.,0.));
#14101=DIRECTION('ref_axis',(0.,0.,-1.));
#14102=DIRECTION('',(1.,0.,0.));
#14103=DIRECTION('center_axis',(1.,0.,-2.52323414687536E-15));
#14104=DIRECTION('ref_axis',(-2.52323414687536E-15,0.,-1.));
#14105=DIRECTION('center_axis',(1.,0.,0.));
#14106=DIRECTION('ref_axis',(0.,0.,-1.));
#14107=DIRECTION('',(1.,0.,0.));
#14108=DIRECTION('center_axis',(-0.991582480911615,3.94488230498385E-15,
0.129476575291316));
#14109=DIRECTION('ref_axis',(0.129476575291316,-1.79884483303906E-11,0.991582480911614));
#14110=DIRECTION('center_axis',(-0.991582480911611,3.9101256326932E-16,
0.12947657529134));
#14111=DIRECTION('ref_axis',(0.12947657529134,-8.50893575937157E-12,0.991582480911611));
#14112=DIRECTION('center_axis',(0.,0.,-1.));
#14113=DIRECTION('ref_axis',(-1.,0.,0.));
#14114=DIRECTION('',(0.,-1.,0.));
#14115=DIRECTION('',(-1.,0.,0.));
#14116=DIRECTION('',(0.,-1.,0.));
#14117=DIRECTION('center_axis',(0.,0.,-1.));
#14118=DIRECTION('ref_axis',(-1.,0.,0.));
#14119=DIRECTION('',(0.,1.,0.));
#14120=DIRECTION('',(-1.,0.,0.));
#14121=DIRECTION('',(0.,1.,0.));
#14122=DIRECTION('center_axis',(1.,0.,-2.52323414687536E-15));
#14123=DIRECTION('ref_axis',(-2.52323414687536E-15,0.,-1.));
#14124=DIRECTION('',(0.,-1.,0.));
#14125=DIRECTION('',(-2.52323414687536E-15,0.,-1.));
#14126=DIRECTION('center_axis',(-1.,0.,2.52323414687536E-15));
#14127=DIRECTION('ref_axis',(-2.52323414687536E-15,0.,-1.));
#14128=DIRECTION('center_axis',(-0.991582480911614,0.,0.129476575291322));
#14129=DIRECTION('ref_axis',(0.129476575291322,0.,0.991582480911614));
#14130=DIRECTION('',(0.129476575291322,0.,0.991582480911614));
#14131=DIRECTION('',(0.,-1.,0.));
#14132=DIRECTION('center_axis',(0.991582480911629,9.22717350759991E-14,
-0.129476575291207));
#14133=DIRECTION('ref_axis',(0.129476575291207,3.62398433939346E-12,0.991582480911629));
#14134=DIRECTION('center_axis',(0.,0.,-1.));
#14135=DIRECTION('ref_axis',(1.,0.,0.));
#14136=DIRECTION('center_axis',(0.,0.,1.));
#14137=DIRECTION('ref_axis',(-1.,-1.38777878078144E-14,0.));
#14138=DIRECTION('',(-1.,0.,0.));
#14139=DIRECTION('center_axis',(0.,0.,1.));
#14140=DIRECTION('ref_axis',(-1.,-1.38777878078144E-14,0.));
#14141=DIRECTION('center_axis',(0.,0.,-1.));
#14142=DIRECTION('ref_axis',(-1.,0.,0.));
#14143=DIRECTION('',(0.,-1.,0.));
#14144=DIRECTION('center_axis',(0.,0.,-1.));
#14145=DIRECTION('ref_axis',(-1.,0.,0.));
#14146=DIRECTION('',(-0.948969605928567,-0.315367542755717,0.));
#14147=DIRECTION('',(0.315367542755717,-0.948969605928567,0.));
#14148=DIRECTION('',(0.948969605928568,0.315367542755717,0.));
#14149=DIRECTION('',(-0.946881588720454,0.32158242635789,0.));
#14150=DIRECTION('center_axis',(0.,0.,-1.));
#14151=DIRECTION('ref_axis',(-1.,0.,0.));
#14152=DIRECTION('',(0.,1.,0.));
#14153=DIRECTION('center_axis',(0.,0.,-1.));
#14154=DIRECTION('ref_axis',(-1.,0.,0.));
#14155=DIRECTION('',(1.,0.,0.));
#14156=DIRECTION('center_axis',(0.,0.,1.));
#14157=DIRECTION('ref_axis',(-1.,0.,0.));
#14158=DIRECTION('',(1.,0.,0.));
#14159=DIRECTION('center_axis',(0.,0.,1.));
#14160=DIRECTION('ref_axis',(1.,-3.92466554034205E-11,0.));
#14161=DIRECTION('center_axis',(0.,0.,1.));
#14162=DIRECTION('ref_axis',(1.,0.,0.));
#14163=DIRECTION('',(1.,0.,0.));
#14164=DIRECTION('center_axis',(0.,0.,1.));
#14165=DIRECTION('ref_axis',(1.,0.,0.));
#14166=DIRECTION('',(-1.,0.,0.));
#14167=DIRECTION('center_axis',(0.,0.,1.));
#14168=DIRECTION('ref_axis',(1.,0.,0.));
#14169=DIRECTION('center_axis',(0.,0.,-1.));
#14170=DIRECTION('ref_axis',(1.,0.,0.));
#14171=DIRECTION('',(0.,-1.,0.));
#14172=DIRECTION('center_axis',(0.,0.,-1.));
#14173=DIRECTION('ref_axis',(1.,1.85037170770859E-15,0.));
#14174=DIRECTION('',(-0.948969605928567,-0.315367542755717,0.));
#14175=DIRECTION('center_axis',(0.,0.,1.));
#14176=DIRECTION('ref_axis',(1.,0.,0.));
#14177=DIRECTION('',(0.948969605928567,0.315367542755717,0.));
#14178=DIRECTION('center_axis',(0.,0.,1.));
#14179=DIRECTION('ref_axis',(1.,0.,0.));
#14180=DIRECTION('center_axis',(0.,0.,-1.));
#14181=DIRECTION('ref_axis',(1.,0.,0.));
#14182=DIRECTION('center_axis',(0.,0.,-1.));
#14183=DIRECTION('ref_axis',(1.,3.60822483003176E-15,0.));
#14184=DIRECTION('',(-0.946881588720454,0.32158242635789,0.));
#14185=DIRECTION('center_axis',(0.,0.,-1.));
#14186=DIRECTION('ref_axis',(1.,9.25185853854296E-16,0.));
#14187=DIRECTION('',(0.,1.,0.));
#14188=DIRECTION('center_axis',(0.,0.,-1.));
#14189=DIRECTION('ref_axis',(1.,0.,0.));
#14190=DIRECTION('center_axis',(0.315367542755717,-0.948969605928568,0.));
#14191=DIRECTION('ref_axis',(0.948969605928567,0.315367542755717,0.));
#14192=DIRECTION('',(-0.948969605928567,-0.315367542755717,0.));
#14193=DIRECTION('',(-1.26920068081332E-33,-4.21788745889624E-34,-1.));
#14194=DIRECTION('',(0.,0.,1.));
#14195=DIRECTION('center_axis',(0.,0.,-1.));
#14196=DIRECTION('ref_axis',(-1.,0.,0.));
#14197=DIRECTION('',(0.,1.,0.));
#14198=DIRECTION('',(1.,0.,0.));
#14199=DIRECTION('',(0.,1.,0.));
#14200=DIRECTION('',(1.,0.,0.));
#14201=DIRECTION('center_axis',(1.,0.,0.));
#14202=DIRECTION('ref_axis',(0.,0.,-1.));
#14203=DIRECTION('center_axis',(1.,0.,0.));
#14204=DIRECTION('ref_axis',(0.,6.93889390390722E-16,1.));
#14205=DIRECTION('',(1.,0.,0.));
#14206=DIRECTION('center_axis',(1.,0.,2.52323414687536E-15));
#14207=DIRECTION('ref_axis',(-2.52323414687536E-15,0.,1.));
#14208=DIRECTION('center_axis',(0.,0.,1.));
#14209=DIRECTION('ref_axis',(1.,0.,0.));
#14210=DIRECTION('center_axis',(0.,0.,-1.));
#14211=DIRECTION('ref_axis',(1.,-1.38777878078144E-14,0.));
#14212=DIRECTION('',(1.,0.,0.));
#14213=DIRECTION('center_axis',(0.,0.,-1.));
#14214=DIRECTION('ref_axis',(1.,-1.38777878078144E-14,0.));
#14215=DIRECTION('',(1.,0.,0.));
#14216=DIRECTION('center_axis',(0.,0.,1.));
#14217=DIRECTION('ref_axis',(1.,0.,0.));
#14218=DIRECTION('',(0.,1.,0.));
#14219=DIRECTION('center_axis',(0.,0.,1.));
#14220=DIRECTION('ref_axis',(1.,0.,0.));
#14221=DIRECTION('',(-0.946881588720454,0.32158242635789,0.));
#14222=DIRECTION('center_axis',(0.,0.,1.));
#14223=DIRECTION('ref_axis',(1.,0.,0.));
#14224=DIRECTION('',(-0.948969605928568,-0.315367542755717,0.));
#14225=DIRECTION('',(-0.315367542755717,0.948969605928567,0.));
#14226=DIRECTION('center_axis',(0.,0.,-1.));
#14227=DIRECTION('ref_axis',(1.,1.54197642309049E-14,0.));
#14228=DIRECTION('center_axis',(0.,0.,1.));
#14229=DIRECTION('ref_axis',(1.,0.,0.));
#14230=DIRECTION('',(0.,-1.,0.));
#14231=DIRECTION('center_axis',(0.,0.,1.));
#14232=DIRECTION('ref_axis',(1.,0.,0.));
#14233=DIRECTION('',(0.,-1.,0.));
#14234=DIRECTION('center_axis',(0.,0.,-1.));
#14235=DIRECTION('ref_axis',(1.,0.,0.));
#14236=DIRECTION('',(1.,0.,0.));
#14237=DIRECTION('center_axis',(0.,0.,-1.));
#14238=DIRECTION('ref_axis',(1.,-5.03906675906735E-11,0.));
#14239=DIRECTION('',(0.,-1.,0.));
#14240=DIRECTION('',(1.,0.,0.));
#14241=DIRECTION('center_axis',(1.,0.,0.));
#14242=DIRECTION('ref_axis',(0.,0.,-1.));
#14243=DIRECTION('',(0.,0.,1.));
#14244=DIRECTION('',(0.,0.,-1.));
#14245=DIRECTION('center_axis',(0.,1.,0.));
#14246=DIRECTION('ref_axis',(0.,0.,1.));
#14247=DIRECTION('',(0.,0.,-1.));
#14248=DIRECTION('',(0.,0.,1.));
#14249=DIRECTION('center_axis',(-1.,0.,0.));
#14250=DIRECTION('ref_axis',(0.,0.,1.));
#14251=DIRECTION('',(0.,0.,-1.));
#14252=DIRECTION('',(0.,0.,1.));
#14253=DIRECTION('center_axis',(-0.32158242635789,-0.946881588720455,0.));
#14254=DIRECTION('ref_axis',(0.946881588720455,-0.32158242635789,0.));
#14255=DIRECTION('',(0.,0.,-1.));
#14256=DIRECTION('',(0.,0.,1.));
#14257=DIRECTION('center_axis',(0.,0.,1.));
#14258=DIRECTION('ref_axis',(1.,0.,0.));
#14259=DIRECTION('center_axis',(-1.,0.,-2.52323414687536E-15));
#14260=DIRECTION('ref_axis',(-2.52323414687536E-15,0.,1.));
#14261=DIRECTION('',(0.,-1.,0.));
#14262=DIRECTION('',(2.52323414687536E-15,0.,-1.));
#14263=DIRECTION('center_axis',(-1.,0.,-2.52323414687536E-15));
#14264=DIRECTION('ref_axis',(-2.52323414687536E-15,0.,1.));
#14265=DIRECTION('',(-2.41889050778795E-15,0.28459828842631,0.958646866278097));
#14266=DIRECTION('center_axis',(0.,-1.,0.));
#14267=DIRECTION('ref_axis',(-0.0648749531344179,0.,0.997893401348965));
#14268=DIRECTION('',(0.,-1.,0.));
#14269=DIRECTION('center_axis',(0.,-1.,0.));
#14270=DIRECTION('ref_axis',(0.,0.,-1.));
#14271=DIRECTION('center_axis',(-1.96841463568603E-16,0.958646866278096,
-0.284598288426311));
#14272=DIRECTION('ref_axis',(6.29350215176821E-14,0.284598288426311,0.958646866278096));
#14273=DIRECTION('center_axis',(0.991582480911614,0.,0.129476575291322));
#14274=DIRECTION('ref_axis',(0.129476575291322,0.,-0.991582480911614));
#14275=DIRECTION('',(-0.129476575291322,0.,0.991582480911614));
#14276=DIRECTION('',(0.124206667879909,-0.28239446456039,-0.95122345957184));
#14277=DIRECTION('center_axis',(-0.991582480911612,3.71896393509484E-15,
-0.129476575291335));
#14278=DIRECTION('ref_axis',(0.129476575291335,-1.65123794436265E-11,-0.991582480911612));
#14279=DIRECTION('',(0.,-1.,0.));
#14280=DIRECTION('center_axis',(0.991582480911607,-7.77925334389506E-14,
0.129476575291374));
#14281=DIRECTION('ref_axis',(0.129476575291374,-9.20853362991702E-11,-0.991582480911607));
#14282=DIRECTION('center_axis',(0.,-1.,0.));
#14283=DIRECTION('ref_axis',(0.,0.,-1.));
#14284=DIRECTION('center_axis',(0.,1.,0.));
#14285=DIRECTION('ref_axis',(0.,0.,-1.));
#14286=DIRECTION('',(0.129476575291322,0.,-0.991582480911614));
#14287=DIRECTION('',(-2.52323414687536E-15,0.,1.));
#14288=DIRECTION('center_axis',(0.,0.,-1.));
#14289=DIRECTION('ref_axis',(-1.,0.,0.));
#14290=DIRECTION('',(0.,-1.,0.));
#14291=DIRECTION('',(1.,0.,0.));
#14292=DIRECTION('',(1.,0.,0.));
#14293=DIRECTION('center_axis',(1.,0.,0.));
#14294=DIRECTION('ref_axis',(0.,0.,-1.));
#14295=DIRECTION('',(1.,0.,0.));
#14296=DIRECTION('center_axis',(-0.991582480911613,7.99403462683938E-16,
-0.129476575291326));
#14297=DIRECTION('ref_axis',(0.129476575291326,-1.62736358106788E-11,-0.991582480911613));
#14298=DIRECTION('center_axis',(0.,0.958646866278097,-0.28459828842631));
#14299=DIRECTION('ref_axis',(0.,0.28459828842631,0.958646866278097));
#14300=DIRECTION('',(0.,0.28459828842631,0.958646866278097));
#14301=DIRECTION('center_axis',(-5.40194110194962E-16,0.958646866278097,
-0.28459828842631));
#14302=DIRECTION('ref_axis',(-5.49346011511301E-14,0.28459828842631,0.958646866278097));
#14303=DIRECTION('',(0.124206667879908,-0.28239446456039,-0.95122345957184));
#14304=DIRECTION('center_axis',(0.,-1.,0.));
#14305=DIRECTION('ref_axis',(0.,0.,-1.));
#14306=DIRECTION('',(-0.129476575291321,0.,0.991582480911614));
#14307=DIRECTION('center_axis',(0.,-1.,0.));
#14308=DIRECTION('ref_axis',(0.,0.,-1.));
#14309=DIRECTION('',(0.,0.,-1.));
#14310=DIRECTION('',(0.99997906305609,0.,-0.00647096974680808));
#14311=DIRECTION('center_axis',(-1.,0.,0.));
#14312=DIRECTION('ref_axis',(0.,0.,1.));
#14313=DIRECTION('center_axis',(1.,0.,0.));
#14314=DIRECTION('ref_axis',(0.,0.,1.));
#14315=DIRECTION('',(0.,1.,0.));
#14316=DIRECTION('',(0.,0.,1.));
#14317=DIRECTION('',(0.,-1.,0.));
#14318=DIRECTION('center_axis',(0.,-1.,0.));
#14319=DIRECTION('ref_axis',(-0.0648749531344181,0.,0.997893401348965));
#14320=DIRECTION('center_axis',(0.,1.,0.));
#14321=DIRECTION('ref_axis',(0.,0.,-1.));
#14322=DIRECTION('',(0.,-1.,0.));
#14323=DIRECTION('center_axis',(0.991582480911614,0.,0.129476575291321));
#14324=DIRECTION('ref_axis',(0.129476575291321,0.,-0.991582480911614));
#14325=DIRECTION('center_axis',(-0.991582480911602,-5.10163316335803E-15,
-0.129476575291414));
#14326=DIRECTION('ref_axis',(0.129476575291414,-9.29749157779182E-11,-0.991582480911602));
#14327=DIRECTION('',(0.129476575291321,0.,-0.991582480911614));
#14328=DIRECTION('',(0.,-1.,0.));
#14329=DIRECTION('center_axis',(-0.00647096974680808,0.,-0.99997906305609));
#14330=DIRECTION('ref_axis',(-0.99997906305609,0.,0.00647096974680808));
#14331=DIRECTION('',(0.99997906305609,0.,-0.00647096974680808));
#14332=DIRECTION('',(0.,1.,0.));
#14333=DIRECTION('',(-0.99997906305609,0.,0.00647096974680808));
#14334=DIRECTION('',(0.,-1.,0.));
#14335=DIRECTION('center_axis',(0.,0.,-1.));
#14336=DIRECTION('ref_axis',(-1.,0.,0.));
#14337=DIRECTION('',(0.,0.,1.));
#14338=DIRECTION('center_axis',(0.671022843491264,0.222998528051552,0.707106781186364));
#14339=DIRECTION('ref_axis',(0.671022847566698,0.222998515787032,-0.707106781186732));
#14340=DIRECTION('center_axis',(0.,0.,-1.));
#14341=DIRECTION('ref_axis',(1.,2.48412401759879E-14,0.));
#14342=DIRECTION('center_axis',(0.,0.,-1.));
#14343=DIRECTION('ref_axis',(-1.,0.,0.));
#14344=DIRECTION('center_axis',(0.,0.,-1.));
#14345=DIRECTION('ref_axis',(-1.,0.,0.));
#14346=DIRECTION('center_axis',(0.,0.,-1.));
#14347=DIRECTION('ref_axis',(-1.,0.,0.));
#14348=DIRECTION('center_axis',(0.,0.,-1.));
#14349=DIRECTION('ref_axis',(-1.,0.,0.));
#14350=DIRECTION('center_axis',(-5.39737656850081E-17,-1.79369009829332E-17,
-1.));
#14351=DIRECTION('ref_axis',(-1.,0.,5.39737656850081E-17));
#14352=DIRECTION('',(0.948969605928567,0.315367542755717,-5.68761795402233E-17));
#14353=DIRECTION('',(0.315367542755717,-0.948969605928567,0.));
#14354=DIRECTION('',(0.948969605928567,0.315367542755717,-5.68761795402233E-17));
#14355=DIRECTION('',(-0.315367542755717,0.948969605928567,3.08148791101958E-33));
#14356=DIRECTION('center_axis',(-0.315367542755717,0.948969605928568,2.77555756156289E-17));
#14357=DIRECTION('ref_axis',(-0.948969605928567,-0.315367542755717,0.));
#14358=DIRECTION('',(0.671022843492016,0.222998528048706,0.707106781186548));
#14359=DIRECTION('',(0.948969605928567,0.315367542755717,0.));
#14360=DIRECTION('',(0.671022843492016,0.222998528048706,-0.707106781186547));
#14361=DIRECTION('center_axis',(0.315367542755717,-0.948969605928567,-2.77555756156289E-17));
#14362=DIRECTION('ref_axis',(-0.948969605928567,-0.315367542755718,1.54074395550979E-33));
#14363=DIRECTION('center_axis',(0.315367542755717,-0.948969605928567,-2.77555756156289E-17));
#14364=DIRECTION('ref_axis',(-0.948969605928567,-0.315367542755718,2.09476042382105E-15));
#14365=DIRECTION('center_axis',(0.671022843492016,0.222998528048706,-0.707106781186547));
#14366=DIRECTION('ref_axis',(-0.725372545860843,-1.38777878078145E-17,-0.688356498996966));
#14367=DIRECTION('',(0.671022843492016,0.222998528048706,0.707106781186548));
#14368=DIRECTION('center_axis',(0.671022843492036,0.222998528048696,-0.707106781186532));
#14369=DIRECTION('ref_axis',(0.671022843491931,0.222998528048912,0.707106781186563));
#14370=DIRECTION('',(-0.315367542755717,0.948969605928567,-9.8130778667736E-18));
#14371=DIRECTION('center_axis',(-0.948969605928568,-0.315367542755717,1.33745135026891E-33));
#14372=DIRECTION('ref_axis',(0.315367542755717,-0.948969605928567,0.));
#14373=DIRECTION('',(0.315367542755717,-0.948969605928567,0.));
#14374=DIRECTION('',(-1.26920068081332E-33,-4.21788745889624E-34,-1.));
#14375=DIRECTION('center_axis',(0.948969605928568,0.315367542755717,-1.33745135026891E-33));
#14376=DIRECTION('ref_axis',(0.315367542755717,-0.948969605928567,1.38777878078145E-14));
#14377=DIRECTION('',(-8.7532076796714E-18,2.63391976542839E-17,-1.));
#14378=DIRECTION('center_axis',(-0.671022843492015,-0.222998528048706,-0.707106781186548));
#14379=DIRECTION('ref_axis',(-0.725372545860843,-2.77555756156289E-17,0.688356498996965));
#14380=DIRECTION('',(0.671022843492016,0.222998528048706,-0.707106781186547));
#14381=DIRECTION('',(0.315367542755717,-0.948969605928567,-2.65650496374544E-17));
#14382=DIRECTION('center_axis',(-0.671022843492001,-0.222998528048843,-0.707106781186518));
#14383=DIRECTION('ref_axis',(0.671022843489952,0.222998528054823,-0.707106781186577));
#14384=DIRECTION('center_axis',(-0.671022843492014,-0.222998528048677,-0.707106781186559));
#14385=DIRECTION('ref_axis',(0.671022843491969,0.222998528048881,-0.707106781186537));
#14386=DIRECTION('center_axis',(-0.315367542755717,0.948969605928568,2.77555756156289E-17));
#14387=DIRECTION('ref_axis',(-0.948969605928567,-0.315367542755717,0.));
#14388=DIRECTION('',(-0.948969605928567,-0.315367542755717,0.));
#14389=DIRECTION('',(8.7532076796714E-18,-2.63391976542839E-17,1.));
#14390=DIRECTION('center_axis',(-0.315367542755717,0.948969605928567,2.77555756156289E-17));
#14391=DIRECTION('ref_axis',(-0.948969605928568,-0.315367542755717,7.70371977754894E-33));
#14392=DIRECTION('center_axis',(-0.315367542755717,0.948969605928567,2.77555756156289E-17));
#14393=DIRECTION('ref_axis',(-0.948969605928567,-0.315367542755718,1.54074395550979E-33));
#14394=DIRECTION('center_axis',(0.,0.,-1.));
#14395=DIRECTION('ref_axis',(-1.,0.,0.));
#14396=DIRECTION('center_axis',(0.,0.,-1.));
#14397=DIRECTION('ref_axis',(-1.,0.,0.));
#14398=DIRECTION('center_axis',(0.,0.,-1.));
#14399=DIRECTION('ref_axis',(-1.,0.,0.));
#14400=DIRECTION('center_axis',(-1.,0.,0.));
#14401=DIRECTION('ref_axis',(0.,0.,1.));
#14402=DIRECTION('',(0.,0.,1.));
#14403=DIRECTION('',(0.,-1.,0.));
#14404=DIRECTION('',(0.,0.,-1.));
#14405=DIRECTION('center_axis',(-0.315367542755717,0.948969605928568,0.));
#14406=DIRECTION('ref_axis',(-0.948969605928567,-0.315367542755717,0.));
#14407=DIRECTION('',(-0.948969605928567,-0.315367542755717,0.));
#14408=DIRECTION('',(0.,0.,1.));
#14409=DIRECTION('center_axis',(0.32158242635789,0.946881588720455,0.));
#14410=DIRECTION('ref_axis',(-0.946881588720455,0.32158242635789,0.));
#14411=DIRECTION('',(-0.946881588720454,0.32158242635789,0.));
#14412=DIRECTION('',(0.,0.,-1.));
#14413=DIRECTION('center_axis',(1.,0.,0.));
#14414=DIRECTION('ref_axis',(0.,0.,-1.));
#14415=DIRECTION('',(0.,1.,0.));
#14416=DIRECTION('',(0.,0.,-1.));
#14417=DIRECTION('',(0.,0.,1.));
#14418=DIRECTION('center_axis',(0.,0.,-1.));
#14419=DIRECTION('ref_axis',(1.,0.,0.));
#14420=DIRECTION('center_axis',(0.,0.,-1.));
#14421=DIRECTION('ref_axis',(-1.,0.,0.));
#14422=DIRECTION('',(1.,0.,0.));
#14423=DIRECTION('center_axis',(0.,0.,-1.));
#14424=DIRECTION('ref_axis',(-1.,0.,0.));
#14425=DIRECTION('center_axis',(0.,0.,1.));
#14426=DIRECTION('ref_axis',(-1.,0.,0.));
#14427=DIRECTION('center_axis',(0.,0.,1.));
#14428=DIRECTION('ref_axis',(-1.,0.,0.));
#14429=DIRECTION('center_axis',(0.,0.,-1.));
#14430=DIRECTION('ref_axis',(-1.,0.,0.));
#14431=DIRECTION('',(-0.948969605928567,-0.315367542755717,0.));
#14432=DIRECTION('center_axis',(0.,0.,1.));
#14433=DIRECTION('ref_axis',(-1.,-9.25185853854296E-16,0.));
#14434=DIRECTION('center_axis',(0.,0.,1.));
#14435=DIRECTION('ref_axis',(-1.,0.,0.));
#14436=DIRECTION('center_axis',(0.,0.,-1.));
#14437=DIRECTION('ref_axis',(1.,0.,0.));
#14438=DIRECTION('center_axis',(0.,-1.,0.));
#14439=DIRECTION('ref_axis',(0.,0.,1.));
#14440=DIRECTION('',(-0.129476575291322,0.,-0.991582480911614));
#14441=DIRECTION('',(2.52323414687536E-15,0.,1.));
#14442=DIRECTION('center_axis',(0.00647096974680808,0.,-0.99997906305609));
#14443=DIRECTION('ref_axis',(-0.99997906305609,0.,-0.00647096974680808));
#14444=DIRECTION('',(-0.99997906305609,0.,-0.00647096974680808));
#14445=DIRECTION('',(0.99997906305609,0.,0.00647096974680808));
#14446=DIRECTION('',(0.,1.,0.));
#14447=DIRECTION('center_axis',(0.00647096974627404,-2.69158824529299E-10,
-0.999979063056094));
#14448=DIRECTION('ref_axis',(-0.00333013267216393,0.999994454860619,-2.1549908119201E-5));
#14449=DIRECTION('center_axis',(1.,0.,0.));
#14450=DIRECTION('ref_axis',(0.,0.,-1.));
#14451=DIRECTION('center_axis',(1.,0.,0.));
#14452=DIRECTION('ref_axis',(0.,0.,-1.));
#14453=DIRECTION('',(0.,0.,1.));
#14454=DIRECTION('',(0.,-1.,0.));
#14455=DIRECTION('center_axis',(-0.991582480911613,0.,0.129476575291326));
#14456=DIRECTION('ref_axis',(0.129476575291326,0.,0.991582480911613));
#14457=DIRECTION('center_axis',(-0.991582480911623,-1.21982113180531E-13,
0.129476575291247));
#14458=DIRECTION('ref_axis',(0.129476575291247,3.37745991995288E-11,0.991582480911624));
#14459=DIRECTION('',(-0.129476575291326,0.,-0.991582480911613));
#14460=DIRECTION('center_axis',(0.,-1.,0.));
#14461=DIRECTION('ref_axis',(0.,0.,-1.));
#14462=DIRECTION('',(0.129476575291326,0.,0.991582480911613));
#14463=DIRECTION('',(0.,0.,-1.));
#14464=DIRECTION('center_axis',(0.,0.,1.));
#14465=DIRECTION('ref_axis',(1.,0.,0.));
#14466=DIRECTION('center_axis',(0.,0.,1.));
#14467=DIRECTION('ref_axis',(1.,0.,0.));
#14468=DIRECTION('center_axis',(0.,0.,1.));
#14469=DIRECTION('ref_axis',(1.,0.,0.));
#14470=DIRECTION('center_axis',(0.,0.,1.));
#14471=DIRECTION('ref_axis',(1.,0.,0.));
#14472=DIRECTION('center_axis',(0.948969605928568,0.315367542755717,1.33745135026891E-33));
#14473=DIRECTION('ref_axis',(-0.315367542755717,0.948969605928567,0.));
#14474=DIRECTION('center_axis',(0.948969605928568,0.315367542755717,1.33745135026891E-33));
#14475=DIRECTION('ref_axis',(-0.315367542755717,0.948969605928567,1.28292706084425E-48));
#14476=DIRECTION('',(1.26920068081332E-33,4.21788745889624E-34,-1.));
#14477=DIRECTION('',(0.315367542755717,-0.948969605928567,0.));
#14478=DIRECTION('',(-8.7532076796714E-18,2.63391976542839E-17,1.));
#14479=DIRECTION('center_axis',(0.671022843492015,0.222998528048706,-0.707106781186548));
#14480=DIRECTION('ref_axis',(-0.725372545860843,-2.77555756156289E-17,-0.688356498996965));
#14481=DIRECTION('',(-0.315367542755717,0.948969605928567,-2.65650496374544E-17));
#14482=DIRECTION('',(0.671022843492016,0.222998528048706,0.707106781186547));
#14483=DIRECTION('center_axis',(-0.671022843492013,-0.222998528048675,0.70710678118656));
#14484=DIRECTION('ref_axis',(0.671022843492034,0.22299852804869,0.707106781186535));
#14485=DIRECTION('center_axis',(-0.671022843491897,-0.222998528049469,0.70710678118642));
#14486=DIRECTION('ref_axis',(0.671022843488484,0.222998528058928,0.707106781186675));
#14487=DIRECTION('center_axis',(5.39737656850081E-17,1.79369009829332E-17,
-1.));
#14488=DIRECTION('ref_axis',(-1.,0.,-5.39737656850081E-17));
#14489=DIRECTION('',(-0.315367542755717,0.948969605928567,0.));
#14490=DIRECTION('',(0.948969605928567,0.315367542755717,5.68761795402233E-17));
#14491=DIRECTION('',(0.315367542755717,-0.948969605928567,3.08148791101958E-33));
#14492=DIRECTION('center_axis',(-0.671022843492016,-0.222998528048706,-0.707106781186547));
#14493=DIRECTION('ref_axis',(-0.725372545860843,-1.38777878078145E-17,0.688356498996966));
#14494=DIRECTION('',(0.671022843492016,0.222998528048706,-0.707106781186548));
#14495=DIRECTION('',(0.315367542755717,-0.948969605928568,-9.8130778667736E-18));
#14496=DIRECTION('center_axis',(0.67102284349202,0.22299852804872,0.70710678118654));
#14497=DIRECTION('ref_axis',(0.671022843491547,0.222998528050093,-0.707106781186555));
#14498=DIRECTION('center_axis',(-0.315367542755717,0.948969605928568,-2.77555756156289E-17));
#14499=DIRECTION('ref_axis',(-0.948969605928567,-0.315367542755717,0.));
#14500=DIRECTION('',(0.948969605928567,0.315367542755717,0.));
#14501=DIRECTION('center_axis',(-0.315367542755717,0.948969605928567,-2.77555756156289E-17));
#14502=DIRECTION('ref_axis',(-0.948969605928567,-0.315367542755718,-1.54074395550979E-33));
#14503=DIRECTION('center_axis',(-0.315367542755717,0.948969605928567,-2.77555756156289E-17));
#14504=DIRECTION('ref_axis',(-0.948969605928567,-0.315367542755718,-1.54074395550979E-33));
#14505=DIRECTION('center_axis',(0.,0.,1.));
#14506=DIRECTION('ref_axis',(-1.,0.,0.));
#14507=DIRECTION('center_axis',(0.,0.,1.));
#14508=DIRECTION('ref_axis',(-1.,0.,0.));
#14509=DIRECTION('center_axis',(0.,0.,1.));
#14510=DIRECTION('ref_axis',(-1.,0.,0.));
#14511=DIRECTION('center_axis',(0.,1.,0.));
#14512=DIRECTION('ref_axis',(0.,0.,1.));
#14513=DIRECTION('center_axis',(0.,1.,0.));
#14514=DIRECTION('ref_axis',(0.,0.,1.));
#14515=DIRECTION('center_axis',(0.,1.,0.));
#14516=DIRECTION('ref_axis',(0.,0.,1.));
#14517=DIRECTION('center_axis',(0.,1.,1.38777878078145E-16));
#14518=DIRECTION('ref_axis',(0.,-1.38777878078145E-16,1.));
#14519=DIRECTION('',(0.,-1.38777878078145E-16,1.));
#14520=DIRECTION('',(-1.,0.,0.));
#14521=DIRECTION('',(0.,-1.38777878078145E-16,1.));
#14522=DIRECTION('',(1.,0.,0.));
#14523=DIRECTION('center_axis',(0.,1.,3.85494105772624E-16));
#14524=DIRECTION('ref_axis',(0.,-3.85494105772624E-16,1.));
#14525=DIRECTION('center_axis',(0.,1.,3.85494105772624E-16));
#14526=DIRECTION('ref_axis',(0.,-3.85494105772624E-16,1.));
#14527=DIRECTION('center_axis',(0.,-1.,-1.23908819712629E-16));
#14528=DIRECTION('ref_axis',(0.,1.23908819712629E-16,-1.));
#14529=DIRECTION('',(0.,1.23908819712629E-16,-1.));
#14530=DIRECTION('',(-1.,0.,0.));
#14531=DIRECTION('',(0.,1.23908819712629E-16,-1.));
#14532=DIRECTION('',(1.,0.,0.));
#14533=DIRECTION('center_axis',(1.,0.,0.));
#14534=DIRECTION('ref_axis',(0.,0.,-1.));
#14535=DIRECTION('center_axis',(-1.,0.,0.));
#14536=DIRECTION('ref_axis',(0.,0.,-1.));
#14537=DIRECTION('',(0.,0.,-1.));
#14538=DIRECTION('center_axis',(1.,0.,0.));
#14539=DIRECTION('ref_axis',(0.,0.,-1.));
#14540=DIRECTION('center_axis',(1.,0.,0.));
#14541=DIRECTION('ref_axis',(0.,0.,-1.));
#14542=DIRECTION('',(0.,0.,-1.));
#14543=DIRECTION('center_axis',(-1.,0.,0.));
#14544=DIRECTION('ref_axis',(0.,1.06752213906265E-15,-1.));
#14545=DIRECTION('center_axis',(1.,0.,0.));
#14546=DIRECTION('ref_axis',(0.,0.,-1.));
#14547=DIRECTION('',(0.,0.,1.));
#14548=DIRECTION('center_axis',(1.,0.,0.));
#14549=DIRECTION('ref_axis',(0.,0.,-1.));
#14550=DIRECTION('center_axis',(1.,0.,0.));
#14551=DIRECTION('ref_axis',(0.,0.,-1.));
#14552=DIRECTION('',(0.,0.,1.));
#14553=DIRECTION('center_axis',(-1.,0.,0.));
#14554=DIRECTION('ref_axis',(0.,6.93889390390722E-15,-1.));
#14555=DIRECTION('center_axis',(-1.,0.,0.));
#14556=DIRECTION('ref_axis',(0.,-3.46944695195361E-15,-1.));
#14557=DIRECTION('center_axis',(0.315367542755717,-0.948969605928568,0.));
#14558=DIRECTION('ref_axis',(0.948969605928568,0.315367542755717,0.));
#14559=DIRECTION('center_axis',(0.315367542755717,-0.948969605928568,1.08947049901316E-33));
#14560=DIRECTION('ref_axis',(0.948969605928568,0.315367542755718,1.71056941445901E-49));
#14561=DIRECTION('center_axis',(0.315367542755717,-0.948969605928568,0.));
#14562=DIRECTION('ref_axis',(0.948969605928568,0.315367542755717,0.));
#14563=DIRECTION('center_axis',(0.315367542755717,-0.948969605928568,-2.17894099802631E-33));
#14564=DIRECTION('ref_axis',(0.948969605928568,0.315367542755718,-2.56585412168851E-49));
#14565=DIRECTION('center_axis',(0.,1.,0.));
#14566=DIRECTION('ref_axis',(0.,0.,1.));
#14567=DIRECTION('center_axis',(4.45059470661737E-15,-0.707106781186553,
0.707106781186542));
#14568=DIRECTION('ref_axis',(6.56775678445617E-13,-0.707106781186542,-0.707106781186553));
#14569=DIRECTION('center_axis',(0.,0.,1.));
#14570=DIRECTION('ref_axis',(1.,0.,0.));
#14571=DIRECTION('center_axis',(-0.129476575291326,0.,-0.991582480911613));
#14572=DIRECTION('ref_axis',(-0.991582480911613,0.,0.129476575291326));
#14573=DIRECTION('center_axis',(0.,1.,0.));
#14574=DIRECTION('ref_axis',(0.,0.,1.));
#14575=DIRECTION('center_axis',(0.,-1.,0.));
#14576=DIRECTION('ref_axis',(0.,0.,-1.));
#14577=DIRECTION('center_axis',(0.,1.,0.));
#14578=DIRECTION('ref_axis',(0.749352174952503,0.,-0.662171667993998));
#14579=DIRECTION('center_axis',(0.,-1.,0.));
#14580=DIRECTION('ref_axis',(0.,0.,-1.));
#14581=DIRECTION('center_axis',(-0.99997906305609,0.,0.00647096974680808));
#14582=DIRECTION('ref_axis',(0.00647096974680808,0.,0.99997906305609));
#14583=DIRECTION('center_axis',(0.99997906305609,0.,-0.00647096974680517));
#14584=DIRECTION('ref_axis',(-0.00647096974680517,0.,-0.99997906305609));
#14585=DIRECTION('center_axis',(-0.99997906305609,0.,0.00647096974681905));
#14586=DIRECTION('ref_axis',(0.00647096974681905,0.,0.99997906305609));
#14587=DIRECTION('center_axis',(1.,0.,0.));
#14588=DIRECTION('ref_axis',(0.,0.,1.));
#14589=DIRECTION('center_axis',(0.,0.,-1.));
#14590=DIRECTION('ref_axis',(1.,0.,0.));
#14591=DIRECTION('center_axis',(0.,1.,0.));
#14592=DIRECTION('ref_axis',(0.,0.,-1.));
#14593=DIRECTION('center_axis',(0.129476575291322,-1.7201214080047E-15,
-0.991582480911614));
#14594=DIRECTION('ref_axis',(0.991582480911614,6.93889390390724E-15,0.129476575291322));
#14595=DIRECTION('center_axis',(0.,0.,1.));
#14596=DIRECTION('ref_axis',(1.,0.,0.));
#14597=DIRECTION('center_axis',(0.,0.,-1.));
#14598=DIRECTION('ref_axis',(-1.,0.,0.));
#14599=DIRECTION('center_axis',(0.129476575291321,0.,-0.991582480911614));
#14600=DIRECTION('ref_axis',(-0.991582480911614,0.,-0.129476575291321));
#14601=DIRECTION('center_axis',(0.129476575291322,0.,-0.991582480911614));
#14602=DIRECTION('ref_axis',(-0.991582480911614,0.,-0.129476575291322));
#14603=DIRECTION('center_axis',(0.,-1.,0.));
#14604=DIRECTION('ref_axis',(-0.0648749531344188,0.,0.997893401348965));
#14605=DIRECTION('center_axis',(0.948969605928567,0.315367542755717,0.));
#14606=DIRECTION('ref_axis',(-0.315367542755717,0.948969605928568,0.));
#14607=DIRECTION('center_axis',(0.948969605928567,0.315367542755717,0.));
#14608=DIRECTION('ref_axis',(-0.315367542755717,0.948969605928568,0.));
#14609=DIRECTION('center_axis',(1.,0.,0.));
#14610=DIRECTION('ref_axis',(0.,0.,-1.));
#14611=DIRECTION('center_axis',(1.,0.,0.));
#14612=DIRECTION('ref_axis',(0.,0.,-1.));
#14613=DIRECTION('center_axis',(1.,0.,0.));
#14614=DIRECTION('ref_axis',(0.,0.,-1.));
#14615=DIRECTION('center_axis',(1.,0.,0.));
#14616=DIRECTION('ref_axis',(0.,0.,-1.));
#14617=DIRECTION('center_axis',(-0.948969605928567,-0.315367542755717,0.));
#14618=DIRECTION('ref_axis',(0.315367542755717,-0.948969605928567,0.));
#14619=DIRECTION('center_axis',(-0.948969605928567,-0.315367542755717,0.));
#14620=DIRECTION('ref_axis',(0.315367542755717,-0.948969605928567,0.));
#14621=DIRECTION('center_axis',(1.,0.,0.));
#14622=DIRECTION('ref_axis',(0.,0.,-1.));
#14623=DIRECTION('center_axis',(1.,0.,0.));
#14624=DIRECTION('ref_axis',(0.,0.,-1.));
#14625=DIRECTION('center_axis',(2.52323414687536E-15,0.,1.));
#14626=DIRECTION('ref_axis',(1.,0.,-2.52323414687536E-15));
#14627=DIRECTION('center_axis',(-0.129476575291322,0.,-0.991582480911614));
#14628=DIRECTION('ref_axis',(-0.991582480911614,0.,0.129476575291322));
#14629=DIRECTION('center_axis',(-2.52323414687536E-15,0.,1.));
#14630=DIRECTION('ref_axis',(1.,0.,2.52323414687536E-15));
#14631=DIRECTION('center_axis',(-2.31296463463574E-15,0.,1.));
#14632=DIRECTION('ref_axis',(1.,0.,2.31296463463574E-15));
#14633=DIRECTION('center_axis',(0.,-1.,0.));
#14634=DIRECTION('ref_axis',(-0.0648749531344198,0.,0.997893401348965));
#14635=DIRECTION('center_axis',(0.129476575291322,0.,-0.991582480911614));
#14636=DIRECTION('ref_axis',(-0.991582480911614,0.,-0.129476575291322));
#14637=DIRECTION('center_axis',(0.129476575291322,0.,-0.991582480911614));
#14638=DIRECTION('ref_axis',(-0.991582480911614,0.,-0.129476575291322));
#14639=DIRECTION('center_axis',(0.,0.,-1.));
#14640=DIRECTION('ref_axis',(-1.,0.,0.));
#14641=DIRECTION('center_axis',(0.,0.,1.));
#14642=DIRECTION('ref_axis',(1.,0.,0.));
#14643=DIRECTION('center_axis',(0.,0.,-1.));
#14644=DIRECTION('ref_axis',(-1.,0.,0.));
#14645=DIRECTION('center_axis',(0.,0.,1.));
#14646=DIRECTION('ref_axis',(1.,0.,0.));
#14647=DIRECTION('center_axis',(-1.26920068081332E-33,-4.21788745889624E-34,
-1.));
#14648=DIRECTION('ref_axis',(0.894021371540723,-0.448024315443308,-9.45720919282255E-34));
#14649=DIRECTION('center_axis',(0.,0.,1.));
#14650=DIRECTION('ref_axis',(1.,0.,0.));
#14651=DIRECTION('center_axis',(0.,0.,-1.));
#14652=DIRECTION('ref_axis',(-1.,0.,0.));
#14653=DIRECTION('center_axis',(1.,0.,0.));
#14654=DIRECTION('ref_axis',(0.,0.,-1.));
#14655=DIRECTION('center_axis',(1.,0.,0.));
#14656=DIRECTION('ref_axis',(0.,0.,-1.));
#17421=CARTESIAN_POINT('',(0.,0.,0.));
#17422=CARTESIAN_POINT('Origin',(37.0412526478464,187.739737607039,231.973593133701));
#17423=CARTESIAN_POINT('',(50.0412526478464,187.739737607039,231.973593133701));
#17424=CARTESIAN_POINT('Origin',(37.0412526478464,187.739737607039,231.973593133701));
#17425=CARTESIAN_POINT('',(49.4412526478464,187.739737607039,232.573593133701));
#17426=CARTESIAN_POINT('',(50.0412526478464,187.739737607039,231.973593133701));
#17427=CARTESIAN_POINT('Origin',(37.0412526478464,187.739737607039,232.573593133701));
#17428=CARTESIAN_POINT('Origin',(37.0412526478464,187.739737607039,273.573593133701));
#17429=CARTESIAN_POINT('',(24.0412526478464,187.739737607039,274.173593133701));
#17430=CARTESIAN_POINT('Origin',(37.0412526478464,187.739737607039,274.173593133701));
#17431=CARTESIAN_POINT('',(24.6412526478463,187.739737607039,273.573593133701));
#17432=CARTESIAN_POINT('',(24.6412526478463,187.739737607039,273.573593133701));
#17433=CARTESIAN_POINT('Origin',(37.0412526478464,187.739737607039,273.573593133701));
#17434=CARTESIAN_POINT('Origin',(11.0412526478464,112.739737607039,219.973593133701));
#17435=CARTESIAN_POINT('',(24.0412526478465,112.739737607039,219.973593133701));
#17436=CARTESIAN_POINT('Origin',(11.0412526478464,112.739737607039,219.973593133701));
#17437=CARTESIAN_POINT('',(23.4412526478464,112.739737607039,220.573593133701));
#17438=CARTESIAN_POINT('',(24.0412526478465,112.739737607039,219.973593133701));
#17439=CARTESIAN_POINT('Origin',(11.0412526478464,112.739737607039,220.573593133701));
#17440=CARTESIAN_POINT('Origin',(277.041252647846,78.7397376070391,221.973593133701));
#17441=CARTESIAN_POINT('',(293.041252647846,78.7397376070391,221.973593133701));
#17442=CARTESIAN_POINT('Origin',(277.041252647846,78.7397376070391,221.973593133701));
#17443=CARTESIAN_POINT('',(292.441252647846,78.7397376070391,222.573593133701));
#17444=CARTESIAN_POINT('',(293.041252647846,78.7397376070391,221.973593133701));
#17445=CARTESIAN_POINT('Origin',(277.041252647846,78.7397376070391,222.573593133701));
#17446=CARTESIAN_POINT('Origin',(11.0412526478464,112.739737607039,285.573593133701));
#17447=CARTESIAN_POINT('',(-1.95874735215359,112.739737607039,286.173593133701));
#17448=CARTESIAN_POINT('Origin',(11.0412526478464,112.739737607039,286.173593133701));
#17449=CARTESIAN_POINT('',(-1.35874735215363,112.739737607039,285.573593133701));
#17450=CARTESIAN_POINT('',(-1.35874735215363,112.739737607039,285.573593133701));
#17451=CARTESIAN_POINT('Origin',(11.0412526478464,112.739737607039,285.573593133701));
#17452=CARTESIAN_POINT('Origin',(277.041252647846,78.7397376070391,283.573593133701));
#17453=CARTESIAN_POINT('',(261.041252647846,78.7397376070391,284.173593133701));
#17454=CARTESIAN_POINT('Origin',(277.041252647846,78.7397376070391,284.173593133701));
#17455=CARTESIAN_POINT('',(261.641252647846,78.7397376070391,283.573593133701));
#17456=CARTESIAN_POINT('',(261.641252647846,78.7397376070391,283.573593133701));
#17457=CARTESIAN_POINT('Origin',(277.041252647846,78.7397376070391,283.573593133701));
#17458=CARTESIAN_POINT('Origin',(-260.909689484712,113.464793580191,211.073593133701));
#17459=CARTESIAN_POINT('',(-259.490535542311,109.194430353513,211.073593133701));
#17460=CARTESIAN_POINT('',(-256.639326258033,114.883947522592,211.073593133701));
#17461=CARTESIAN_POINT('Origin',(-260.909689484712,113.464793580191,211.073593133701));
#17462=CARTESIAN_POINT('',(-259.490535542311,109.194430353513,215.573593133701));
#17463=CARTESIAN_POINT('',(-259.490535542311,109.194430353513,211.073593133701));
#17464=CARTESIAN_POINT('',(-257.691868353316,110.319062001314,215.573593133701));
#17465=CARTESIAN_POINT('Origin',(-260.909689484712,113.464793580191,215.573593133701));
#17466=CARTESIAN_POINT('',(-256.639326258033,114.883947522592,211.573593133701));
#17467=CARTESIAN_POINT('Ctrl Pts',(-257.691868353317,110.319062001314,215.573593133701));
#17468=CARTESIAN_POINT('Ctrl Pts',(-257.226722972947,110.794866944168,215.573593133701));
#17469=CARTESIAN_POINT('Ctrl Pts',(-256.875952954917,111.37569206742,215.537123333329));
#17470=CARTESIAN_POINT('Ctrl Pts',(-256.575993830868,112.221556348799,215.307227076609));
#17471=CARTESIAN_POINT('Ctrl Pts',(-256.503984375586,112.507585568265,215.204277782028));
#17472=CARTESIAN_POINT('Ctrl Pts',(-256.419927726647,113.054277491751,214.929717220809));
#17473=CARTESIAN_POINT('Ctrl Pts',(-256.406892655266,113.314450931809,214.75743570919));
#17474=CARTESIAN_POINT('Ctrl Pts',(-256.416576787744,113.953138581935,214.220216585689));
#17475=CARTESIAN_POINT('Ctrl Pts',(-256.482778257329,114.307185871813,213.752911915794));
#17476=CARTESIAN_POINT('Ctrl Pts',(-256.596967428487,114.771542993549,212.703946142401));
#17477=CARTESIAN_POINT('Ctrl Pts',(-256.639326258033,114.883947522592,212.122608190933));
#17478=CARTESIAN_POINT('Ctrl Pts',(-256.639326258033,114.883947522592,211.573593133701));
#17479=CARTESIAN_POINT('',(-256.639326258033,114.883947522592,253.073593133701));
#17480=CARTESIAN_POINT('Origin',(203.041252647846,82.7397376070391,167.073593133701));
#17481=CARTESIAN_POINT('',(226.839232189725,88.7397376070391,163.966155326709));
#17482=CARTESIAN_POINT('',(179.041252647846,88.7397376070391,167.073593133701));
#17483=CARTESIAN_POINT('Origin',(203.041252647846,88.7397376070391,167.073593133701));
#17484=CARTESIAN_POINT('',(232.788727075195,82.7397376070391,163.189295874961));
#17485=CARTESIAN_POINT('Origin',(226.839232189725,82.7397376070391,163.966155326709));
#17486=CARTESIAN_POINT('',(173.041252647846,82.7397376070391,167.073593133701));
#17487=CARTESIAN_POINT('Origin',(203.041252647846,82.7397376070391,167.073593133701));
#17488=CARTESIAN_POINT('Origin',(179.041252647846,82.7397376070391,167.073593133701));
#17489=CARTESIAN_POINT('Origin',(277.041252647846,78.7397376070391,288.573593133701));
#17490=CARTESIAN_POINT('',(259.041252647846,78.7397376070391,290.573593133701));
#17491=CARTESIAN_POINT('Origin',(277.041252647846,78.7397376070391,290.573593133701));
#17492=CARTESIAN_POINT('',(261.041252647846,78.7397376070391,288.573593133701));
#17493=CARTESIAN_POINT('Origin',(259.041252647846,78.7397376070391,288.573593133701));
#17494=CARTESIAN_POINT('Origin',(277.041252647846,78.7397376070391,288.573593133701));
#17495=CARTESIAN_POINT('Origin',(11.0412526478464,112.739737607039,288.573593133701));
#17496=CARTESIAN_POINT('',(-3.95874735215359,112.739737607039,290.573593133701));
#17497=CARTESIAN_POINT('Origin',(11.0412526478464,112.739737607039,290.573593133701));
#17498=CARTESIAN_POINT('',(-1.95874735215359,112.739737607039,288.573593133701));
#17499=CARTESIAN_POINT('Origin',(-3.95874735215359,112.739737607039,288.573593133701));
#17500=CARTESIAN_POINT('Origin',(11.0412526478464,112.739737607039,288.573593133701));
#17501=CARTESIAN_POINT('Origin',(11.0412526478464,112.739737607039,217.573593133701));
#17502=CARTESIAN_POINT('',(26.0412526478465,112.739737607039,215.573593133701));
#17503=CARTESIAN_POINT('Origin',(11.0412526478464,112.739737607039,215.573593133701));
#17504=CARTESIAN_POINT('',(24.0412526478465,112.739737607039,217.573593133701));
#17505=CARTESIAN_POINT('Origin',(26.0412526478465,112.739737607039,217.573593133701));
#17506=CARTESIAN_POINT('Origin',(11.0412526478464,112.739737607039,217.573593133701));
#17507=CARTESIAN_POINT('Origin',(277.041252647846,78.7397376070391,217.573593133701));
#17508=CARTESIAN_POINT('',(295.041252647846,78.7397376070391,215.573593133701));
#17509=CARTESIAN_POINT('Origin',(277.041252647846,78.7397376070391,215.573593133701));
#17510=CARTESIAN_POINT('',(293.041252647846,78.7397376070391,217.573593133701));
#17511=CARTESIAN_POINT('Origin',(295.041252647846,78.7397376070391,217.573593133701));
#17512=CARTESIAN_POINT('Origin',(277.041252647846,78.7397376070391,217.573593133701));
#17513=CARTESIAN_POINT('Origin',(37.0412526478464,187.739737607039,217.573593133701));
#17514=CARTESIAN_POINT('',(41.2239632420135,202.144769092095,215.573593133701));
#17515=CARTESIAN_POINT('',(32.9752147767065,202.178135580168,215.573593133701));
#17516=CARTESIAN_POINT('Origin',(37.0412526478464,187.739737607039,215.573593133701));
#17517=CARTESIAN_POINT('',(40.6662684961245,200.224098227421,217.573593133701));
#17518=CARTESIAN_POINT('Origin',(41.2239632420135,202.144769092095,217.573593133701));
#17519=CARTESIAN_POINT('',(50.0412526478464,187.739737607039,217.573593133701));
#17520=CARTESIAN_POINT('Origin',(37.0412526478464,187.739737607039,217.573593133701));
#17521=CARTESIAN_POINT('',(33.5173531595251,200.253015850418,217.573593133701));
#17522=CARTESIAN_POINT('Origin',(37.0412526478464,187.739737607039,217.573593133701));
#17523=CARTESIAN_POINT('Origin',(32.9752147767065,202.178135580168,217.573593133701));
#17524=CARTESIAN_POINT('Origin',(37.0412526478464,187.739737607039,288.573593133701));
#17525=CARTESIAN_POINT('',(32.9752147767065,202.178135580168,290.573593133701));
#17526=CARTESIAN_POINT('',(41.2239632420135,202.144769092095,290.573593133701));
#17527=CARTESIAN_POINT('Origin',(37.0412526478464,187.739737607039,290.573593133701));
#17528=CARTESIAN_POINT('',(33.5173531595251,200.253015850418,288.573593133701));
#17529=CARTESIAN_POINT('Origin',(32.9752147767065,202.178135580168,288.573593133701));
#17530=CARTESIAN_POINT('',(24.0412526478464,187.739737607039,288.573593133701));
#17531=CARTESIAN_POINT('Origin',(37.0412526478464,187.739737607039,288.573593133701));
#17532=CARTESIAN_POINT('',(40.6662684961245,200.224098227421,288.573593133701));
#17533=CARTESIAN_POINT('Origin',(37.0412526478464,187.739737607039,288.573593133701));
#17534=CARTESIAN_POINT('Origin',(41.2239632420135,202.144769092095,288.573593133701));
#17535=CARTESIAN_POINT('Origin',(-276.958747352154,52.7397376070391,288.573593133701));
#17536=CARTESIAN_POINT('',(-288.458747352154,52.7397376070391,290.573593133701));
#17537=CARTESIAN_POINT('Origin',(-276.958747352154,52.7397376070391,290.573593133701));
#17538=CARTESIAN_POINT('',(-286.458747352154,52.7397376070391,288.573593133701));
#17539=CARTESIAN_POINT('Origin',(-288.458747352154,52.7397376070391,288.573593133701));
#17540=CARTESIAN_POINT('',(-267.458747352154,52.7397376070391,288.573593133701));
#17541=CARTESIAN_POINT('Origin',(-276.958747352154,52.7397376070391,288.573593133701));
#17542=CARTESIAN_POINT('Origin',(-276.958747352154,52.7397376070391,288.573593133701));
#17543=CARTESIAN_POINT('Origin',(-276.958747352154,52.7397376070391,217.573593133701));
#17544=CARTESIAN_POINT('',(-265.458747352154,52.7397376070391,215.573593133701));
#17545=CARTESIAN_POINT('Origin',(-276.958747352154,52.7397376070391,215.573593133701));
#17546=CARTESIAN_POINT('',(-267.458747352154,52.7397376070391,217.573593133701));
#17547=CARTESIAN_POINT('Origin',(-265.458747352154,52.7397376070391,217.573593133701));
#17548=CARTESIAN_POINT('Origin',(-276.958747352154,52.7397376070391,217.573593133701));
#17549=CARTESIAN_POINT('Origin',(-276.958747352154,52.7397376070391,297.073593133701));
#17550=CARTESIAN_POINT('',(-267.458747352154,52.7397376070391,297.073593133701));
#17551=CARTESIAN_POINT('',(-286.458747352154,52.7397376070391,297.073593133701));
#17552=CARTESIAN_POINT('Origin',(-276.958747352154,52.7397376070391,297.073593133701));
#17553=CARTESIAN_POINT('Origin',(-276.958747352154,52.7397376070391,297.073593133701));
#17554=CARTESIAN_POINT('',(-288.458747352154,52.7397376070391,295.073593133701));
#17555=CARTESIAN_POINT('Origin',(-288.458747352154,52.7397376070391,297.073593133701));
#17556=CARTESIAN_POINT('Origin',(-276.958747352154,52.7397376070391,295.073593133701));
#17557=CARTESIAN_POINT('Origin',(-276.958747352154,52.7397376070391,209.073593133701));
#17558=CARTESIAN_POINT('',(-286.458747352154,52.7397376070391,209.073593133701));
#17559=CARTESIAN_POINT('',(-267.458747352154,52.7397376070391,209.073593133701));
#17560=CARTESIAN_POINT('Origin',(-276.958747352154,52.7397376070391,209.073593133701));
#17561=CARTESIAN_POINT('Origin',(-276.958747352154,52.7397376070391,209.073593133701));
#17562=CARTESIAN_POINT('',(-265.458747352154,52.7397376070391,211.073593133701));
#17563=CARTESIAN_POINT('Origin',(-265.458747352154,52.7397376070391,209.073593133701));
#17564=CARTESIAN_POINT('Origin',(-276.958747352154,52.7397376070391,211.073593133701));
#17565=CARTESIAN_POINT('Origin',(231.506382410955,182.009983898606,207.432430075574));
#17566=CARTESIAN_POINT('',(231.480498531968,37.7397376070391,211.432346327798));
#17567=CARTESIAN_POINT('',(233.162260300213,37.7397376070391,211.073593133701));
#17568=CARTESIAN_POINT('Origin',(231.506382410955,37.7397376070391,207.432430075574));
#17569=CARTESIAN_POINT('',(231.480498531968,85.7397376070391,211.432346327798));
#17570=CARTESIAN_POINT('',(231.480498531968,37.7397376070391,211.432346327798));
#17571=CARTESIAN_POINT('',(232.024288712121,85.7397376070391,211.39875999922));
#17572=CARTESIAN_POINT('Origin',(231.506382410955,85.7397376070391,207.432430075574));
#17573=CARTESIAN_POINT('',(235.472712334602,81.7397376070391,206.914523774409));
#17574=CARTESIAN_POINT('Origin',(231.506382410961,81.739737607044,207.432430075578));
#17575=CARTESIAN_POINT('',(235.472712334602,37.7397376070391,206.914523774409));
#17576=CARTESIAN_POINT('',(235.472712334602,85.7397376070391,206.914523774409));
#17577=CARTESIAN_POINT('Origin',(231.506382410955,37.7397376070391,207.432430075574));
#17578=CARTESIAN_POINT('Origin',(203.041252647846,81.7397376070391,167.073593133701));
#17579=CARTESIAN_POINT('',(180.041252647846,85.7397376070391,167.073593133701));
#17580=CARTESIAN_POINT('',(225.847649708814,85.7397376070391,164.095631902));
#17581=CARTESIAN_POINT('Origin',(203.041252647846,85.7397376070391,167.073593133701));
#17582=CARTESIAN_POINT('',(176.041252647846,81.7397376070391,167.073593133701));
#17583=CARTESIAN_POINT('Origin',(180.041252647846,81.7397376070391,167.073593133701));
#17584=CARTESIAN_POINT('',(229.81397963246,81.7397376070391,163.577725600835));
#17585=CARTESIAN_POINT('Origin',(203.041252647846,81.7397376070391,167.073593133701));
#17586=CARTESIAN_POINT('Origin',(225.847649708814,81.7397376070391,164.095631902));
#17587=CARTESIAN_POINT('Origin',(-276.958747352154,52.7397376070391,137.073593133701));
#17588=CARTESIAN_POINT('',(-282.958747352154,52.7397376070391,198.823593133701));
#17589=CARTESIAN_POINT('Origin',(-276.958747352154,52.7397376070391,198.823593133701));
#17590=CARTESIAN_POINT('',(-282.958747352154,52.7397376070391,307.323593133701));
#17591=CARTESIAN_POINT('',(-282.958747352154,52.7397376070391,137.073593133701));
#17592=CARTESIAN_POINT('Origin',(-276.958747352154,52.7397376070391,307.323593133701));
#17593=CARTESIAN_POINT('Origin',(11.0412526478464,112.739737607039,220.573593133701));
#17594=CARTESIAN_POINT('',(24.0412526478465,112.739737607039,220.573593133701));
#17595=CARTESIAN_POINT('Origin',(37.0412526478464,187.739737607039,232.573593133701));
#17596=CARTESIAN_POINT('',(50.0412526478464,187.739737607039,232.573593133701));
#17597=CARTESIAN_POINT('Ctrl Pts',(40.6662684961245,200.224098227421,217.573593133701));
#17598=CARTESIAN_POINT('Ctrl Pts',(40.0831826062374,200.393405703872,217.573593133701));
#17599=CARTESIAN_POINT('Ctrl Pts',(39.4921714450088,200.520958444757,217.554555800012));
#17600=CARTESIAN_POINT('Ctrl Pts',(38.5932073487587,200.650318107912,217.531285607299));
#17601=CARTESIAN_POINT('Ctrl Pts',(38.290917247095,200.68305475883,217.524189505008));
#17602=CARTESIAN_POINT('Ctrl Pts',(37.688803228723,200.727108347403,217.514471384328));
#17603=CARTESIAN_POINT('Ctrl Pts',(37.3882478564454,200.73856950399,217.511826783315));
#17604=CARTESIAN_POINT('Ctrl Pts',(36.4880719422569,200.741819615196,217.511924454037));
#17605=CARTESIAN_POINT('Ctrl Pts',(35.8899421476187,200.7026257403,217.523628183181));
#17606=CARTESIAN_POINT('Ctrl Pts',(34.6975601484818,200.540873888315,217.55445906248));
#17607=CARTESIAN_POINT('Ctrl Pts',(34.101487070175,200.417515444274,217.573593133701));
#17608=CARTESIAN_POINT('Ctrl Pts',(33.5173531595251,200.253015850418,217.573593133701));
#17609=CARTESIAN_POINT('Origin',(277.041252647846,78.7397376070391,222.573593133701));
#17610=CARTESIAN_POINT('',(293.041252647846,78.7397376070391,222.573593133701));
#17611=CARTESIAN_POINT('Origin',(203.041252647846,182.009983898606,167.073593133701));
#17612=CARTESIAN_POINT('',(176.041252647846,70.8334876070391,167.073593133701));
#17613=CARTESIAN_POINT('',(176.041252647846,182.009983898606,167.073593133701));
#17614=CARTESIAN_POINT('',(229.81397963246,71.8713232808586,163.577725600835));
#17615=CARTESIAN_POINT('Origin',(203.041252647847,70.8334876070393,167.0735931337));
#17616=CARTESIAN_POINT('',(229.81397963246,182.009983898606,163.577725600835));
#17617=CARTESIAN_POINT('Origin',(-276.958747352154,52.7397376070391,198.823593133701));
#17618=CARTESIAN_POINT('',(-286.458747352154,52.7397376070391,198.823593133701));
#17619=CARTESIAN_POINT('',(-286.458747352154,52.7397376070391,198.823593133701));
#17620=CARTESIAN_POINT('Origin',(-276.958747352154,52.7397376070391,198.823593133701));
#17621=CARTESIAN_POINT('Origin',(11.0412526478464,112.739737607039,211.073593133701));
#17622=CARTESIAN_POINT('',(5.04125264784645,112.739737607039,211.073593133701));
#17623=CARTESIAN_POINT('Origin',(11.0412526478464,112.739737607039,211.073593133701));
#17624=CARTESIAN_POINT('',(5.04125264784645,112.739737607039,220.573593133701));
#17625=CARTESIAN_POINT('',(5.04125264784645,112.739737607039,211.073593133701));
#17626=CARTESIAN_POINT('Origin',(11.0412526478464,112.739737607039,220.573593133701));
#17627=CARTESIAN_POINT('Origin',(277.041252647846,78.7397376070391,211.073593133701));
#17628=CARTESIAN_POINT('',(269.041252647846,78.7397376070391,211.073593133701));
#17629=CARTESIAN_POINT('Origin',(277.041252647846,78.7397376070391,211.073593133701));
#17630=CARTESIAN_POINT('',(269.041252647846,78.7397376070391,222.573593133701));
#17631=CARTESIAN_POINT('',(269.041252647846,78.7397376070391,211.073593133701));
#17632=CARTESIAN_POINT('Origin',(277.041252647846,78.7397376070391,222.573593133701));
#17633=CARTESIAN_POINT('Origin',(37.0412526478464,187.739737607039,211.073593133701));
#17634=CARTESIAN_POINT('',(29.0412526478464,187.739737607039,211.073593133701));
#17635=CARTESIAN_POINT('Origin',(37.0412526478464,187.739737607039,211.073593133701));
#17636=CARTESIAN_POINT('',(29.0412526478464,187.739737607039,232.573593133701));
#17637=CARTESIAN_POINT('',(29.0412526478464,187.739737607039,211.073593133701));
#17638=CARTESIAN_POINT('Origin',(37.0412526478464,187.739737607039,232.573593133701));
#17639=CARTESIAN_POINT('Origin',(11.0412526478464,112.739737607039,285.573593133701));
#17640=CARTESIAN_POINT('',(-1.95874735215359,112.739737607039,285.573593133701));
#17641=CARTESIAN_POINT('Origin',(37.0412526478464,187.739737607039,273.573593133701));
#17642=CARTESIAN_POINT('',(24.0412526478464,187.739737607039,273.573593133701));
#17643=CARTESIAN_POINT('Ctrl Pts',(33.5173531595251,200.253015850418,288.573593133701));
#17644=CARTESIAN_POINT('Ctrl Pts',(34.1017896558591,200.41760065628,288.573593133701));
#17645=CARTESIAN_POINT('Ctrl Pts',(34.6938133708609,200.540367977988,288.59263046739));
#17646=CARTESIAN_POINT('Ctrl Pts',(35.5937945612941,200.662450841916,288.615900660103));
#17647=CARTESIAN_POINT('Ctrl Pts',(35.896339608343,200.692740912621,288.622996762393));
#17648=CARTESIAN_POINT('Ctrl Pts',(36.4987903139835,200.731921992999,288.632714883073));
#17649=CARTESIAN_POINT('Ctrl Pts',(36.7994285709306,200.740951299452,288.635359484086));
#17650=CARTESIAN_POINT('Ctrl Pts',(37.6996013208751,200.736918934719,288.635261813365));
#17651=CARTESIAN_POINT('Ctrl Pts',(38.2973944661359,200.69288750796,288.62355808422));
#17652=CARTESIAN_POINT('Ctrl Pts',(39.4884288827824,200.521494649736,288.592727204922));
#17653=CARTESIAN_POINT('Ctrl Pts',(40.0834844926596,200.393318046755,288.573593133701));
#17654=CARTESIAN_POINT('Ctrl Pts',(40.6662684961245,200.224098227421,288.573593133701));
#17655=CARTESIAN_POINT('Origin',(277.041252647846,78.7397376070391,283.573593133701));
#17656=CARTESIAN_POINT('',(261.041252647846,78.7397376070391,283.573593133701));
#17657=CARTESIAN_POINT('Origin',(-276.958747352154,52.7397376070391,307.323593133701));
#17658=CARTESIAN_POINT('',(-267.458747352154,52.7397376070391,307.323593133701));
#17659=CARTESIAN_POINT('',(-267.458747352154,52.7397376070391,307.323593133701));
#17660=CARTESIAN_POINT('Origin',(-276.958747352154,52.7397376070391,307.323593133701));
#17661=CARTESIAN_POINT('Origin',(11.0412526478464,112.739737607039,295.073593133701));
#17662=CARTESIAN_POINT('',(17.0412526478464,112.739737607039,295.073593133701));
#17663=CARTESIAN_POINT('Origin',(11.0412526478464,112.739737607039,295.073593133701));
#17664=CARTESIAN_POINT('',(17.0412526478464,112.739737607039,285.573593133701));
#17665=CARTESIAN_POINT('',(17.0412526478464,112.739737607039,295.073593133701));
#17666=CARTESIAN_POINT('Origin',(11.0412526478464,112.739737607039,285.573593133701));
#17667=CARTESIAN_POINT('Origin',(277.041252647846,78.7397376070391,295.073593133701));
#17668=CARTESIAN_POINT('',(285.041252647846,78.7397376070391,295.073593133701));
#17669=CARTESIAN_POINT('Origin',(277.041252647846,78.7397376070391,295.073593133701));
#17670=CARTESIAN_POINT('',(285.041252647846,78.7397376070391,283.573593133701));
#17671=CARTESIAN_POINT('',(285.041252647846,78.7397376070391,295.073593133701));
#17672=CARTESIAN_POINT('Origin',(277.041252647846,78.7397376070391,283.573593133701));
#17673=CARTESIAN_POINT('Origin',(37.0412526478464,187.739737607039,295.073593133701));
#17674=CARTESIAN_POINT('',(45.0412526478464,187.739737607039,295.073593133701));
#17675=CARTESIAN_POINT('Origin',(37.0412526478464,187.739737607039,295.073593133701));
#17676=CARTESIAN_POINT('',(45.0412526478464,187.739737607039,273.573593133701));
#17677=CARTESIAN_POINT('',(45.0412526478464,187.739737607039,295.073593133701));
#17678=CARTESIAN_POINT('Origin',(37.0412526478464,187.739737607039,273.573593133701));
#17679=CARTESIAN_POINT('Origin',(-276.958747352154,52.7397376070391,290.573593133701));
#17680=CARTESIAN_POINT('',(-267.458747352154,52.7397376070391,290.573593133701));
#17681=CARTESIAN_POINT('Origin',(203.041252647846,88.7397376070391,339.073593133701));
#17682=CARTESIAN_POINT('',(203.041252647846,88.7397376070391,344.073593133701));
#17683=CARTESIAN_POINT('Origin',(203.041252647846,88.7397376070391,339.073593133701));
#17684=CARTESIAN_POINT('',(203.041252647846,85.7397376070391,344.073593133701));
#17685=CARTESIAN_POINT('',(203.041252647846,88.7397376070391,344.073593133701));
#17686=CARTESIAN_POINT('Origin',(203.041252647846,85.7397376070391,339.073593133701));
#17687=CARTESIAN_POINT('Origin',(203.041252647846,88.7397376070391,167.073593133701));
#17688=CARTESIAN_POINT('',(232.788727075195,71.9866383557274,163.189295874961));
#17689=CARTESIAN_POINT('',(232.788727075195,88.7397376070391,163.189295874961));
#17690=CARTESIAN_POINT('',(173.041252647846,70.8334876070391,167.073593133701));
#17691=CARTESIAN_POINT('Origin',(203.041252647851,70.8334876070379,167.073593133705));
#17692=CARTESIAN_POINT('',(173.041252647846,88.7397376070391,167.073593133701));
#17693=CARTESIAN_POINT('Origin',(203.041252647846,88.7397376070391,167.073593133701));
#17694=CARTESIAN_POINT('',(203.041252647846,88.7397376070391,172.073593133701));
#17695=CARTESIAN_POINT('Origin',(203.041252647846,88.7397376070391,167.073593133701));
#17696=CARTESIAN_POINT('',(203.041252647846,85.7397376070391,172.073593133701));
#17697=CARTESIAN_POINT('',(203.041252647846,88.7397376070391,172.073593133701));
#17698=CARTESIAN_POINT('Origin',(203.041252647846,85.7397376070391,167.073593133701));
#17699=CARTESIAN_POINT('Origin',(-293.958747352154,37.7397376070391,211.073593133701));
#17700=CARTESIAN_POINT('',(173.041252647846,37.7397376070391,203.073593133701));
#17701=CARTESIAN_POINT('',(173.041252647846,37.7397376070391,211.073593133701));
#17702=CARTESIAN_POINT('',(173.041252647846,37.7397376070391,167.073593133701));
#17703=CARTESIAN_POINT('',(176.041252647846,37.7397376070391,203.073593133701));
#17704=CARTESIAN_POINT('',(-293.958747352154,37.7397376070391,203.073593133701));
#17705=CARTESIAN_POINT('',(176.041252647846,37.7397376070391,207.0993938051));
#17706=CARTESIAN_POINT('',(176.041252647846,37.7397376070391,167.073593133701));
#17707=CARTESIAN_POINT('',(179.587667268292,37.7397376070391,211.073593133701));
#17708=CARTESIAN_POINT('Origin',(180.041252647846,37.7397376070391,207.0993938051));
#17709=CARTESIAN_POINT('',(82.0412526478464,37.7397376070391,211.073593133701));
#17710=CARTESIAN_POINT('Origin',(-293.958747352154,37.7397376070391,211.073593133701));
#17711=CARTESIAN_POINT('',(-278.958747352154,37.7397376070391,211.073593133701));
#17712=CARTESIAN_POINT('',(80.0412526478464,37.7397376070391,211.073593133701));
#17713=CARTESIAN_POINT('',(-293.958747352154,37.7397376070391,211.073593133701));
#17714=CARTESIAN_POINT('',(80.0412526478464,37.7397376070391,215.573593133701));
#17715=CARTESIAN_POINT('',(80.0412526478464,37.7397376070391,211.073593133701));
#17716=CARTESIAN_POINT('',(-278.958747352154,37.7397376070391,215.573593133701));
#17717=CARTESIAN_POINT('',(-293.958747352154,37.7397376070391,215.573593133701));
#17718=CARTESIAN_POINT('',(-278.958747352154,37.7397376070391,211.073593133701));
#17719=CARTESIAN_POINT('Origin',(-293.958747352154,37.7397376070391,211.073593133701));
#17720=CARTESIAN_POINT('',(234.971180132426,37.7397376070391,203.073593133701));
#17721=CARTESIAN_POINT('',(234.760748217833,37.7397376070391,201.462022859575));
#17722=CARTESIAN_POINT('',(237.996647058024,37.7397376070391,203.073593133701));
#17723=CARTESIAN_POINT('',(-293.958747352154,37.7397376070391,203.073593133701));
#17724=CARTESIAN_POINT('',(239.041252647847,37.7397376070391,211.073593133701));
#17725=CARTESIAN_POINT('',(239.041252647847,37.7397376070391,211.073593133701));
#17726=CARTESIAN_POINT('',(82.0412526478464,37.7397376070391,211.073593133701));
#17727=CARTESIAN_POINT('Origin',(-293.958747352154,37.7397376070391,295.073593133701));
#17728=CARTESIAN_POINT('',(176.041252647846,37.7397376070391,303.073593133701));
#17729=CARTESIAN_POINT('',(176.041252647846,37.7397376070391,299.047792462302));
#17730=CARTESIAN_POINT('',(176.041252647846,37.7397376070391,305.073593133701));
#17731=CARTESIAN_POINT('',(173.041252647846,37.7397376070391,303.073593133701));
#17732=CARTESIAN_POINT('',(-293.958747352154,37.7397376070391,303.073593133701));
#17733=CARTESIAN_POINT('',(173.041252647846,37.7397376070391,295.073593133701));
#17734=CARTESIAN_POINT('',(173.041252647846,37.7397376070391,339.073593133701));
#17735=CARTESIAN_POINT('',(179.587667268292,37.7397376070391,295.073593133701));
#17736=CARTESIAN_POINT('',(82.0412526478464,37.7397376070391,295.073593133701));
#17737=CARTESIAN_POINT('Origin',(180.041252647846,37.7397376070391,299.047792462302));
#17738=CARTESIAN_POINT('Origin',(-293.958747352154,37.7397376070391,295.073593133701));
#17739=CARTESIAN_POINT('',(-278.958747352154,37.7397376070391,290.573593133701));
#17740=CARTESIAN_POINT('',(80.0412526478464,37.7397376070391,290.573593133701));
#17741=CARTESIAN_POINT('',(-293.958747352154,37.7397376070391,290.573593133701));
#17742=CARTESIAN_POINT('',(80.0412526478464,37.7397376070391,295.073593133701));
#17743=CARTESIAN_POINT('',(80.0412526478464,37.7397376070391,295.073593133701));
#17744=CARTESIAN_POINT('',(-278.958747352154,37.7397376070391,295.073593133701));
#17745=CARTESIAN_POINT('',(-293.958747352154,37.7397376070391,295.073593133701));
#17746=CARTESIAN_POINT('',(-278.958747352154,37.7397376070391,295.073593133701));
#17747=CARTESIAN_POINT('Origin',(-293.958747352154,37.7397376070391,295.073593133701));
#17748=CARTESIAN_POINT('',(239.041252647847,37.7397376070391,295.073593133701));
#17749=CARTESIAN_POINT('',(237.996647058024,37.7397376070391,303.073593133701));
#17750=CARTESIAN_POINT('',(239.041252647847,37.7397376070391,295.073593133701));
#17751=CARTESIAN_POINT('',(234.971180132426,37.7397376070391,303.073593133701));
#17752=CARTESIAN_POINT('',(-293.958747352154,37.7397376070391,303.073593133701));
#17753=CARTESIAN_POINT('',(235.472712334602,37.7397376070391,299.232662492993));
#17754=CARTESIAN_POINT('',(233.826607434235,37.7397376070391,311.839180523564));
#17755=CARTESIAN_POINT('',(233.162260300213,37.7397376070391,295.073593133701));
#17756=CARTESIAN_POINT('Origin',(231.506382410955,37.7397376070391,298.714756191828));
#17757=CARTESIAN_POINT('',(82.0412526478464,37.7397376070391,295.073593133701));
#17758=CARTESIAN_POINT('Origin',(36.6954328642313,102.247359653123,211.073593133701));
#17759=CARTESIAN_POINT('',(19.2205075843702,200.70865654923,214.922518540102));
#17760=CARTESIAN_POINT('',(14.7441480327787,199.808320566024,210.390652633755));
#17761=CARTESIAN_POINT('Origin',(36.6954317604653,102.24736509754,200.454194907216));
#17762=CARTESIAN_POINT('',(19.2205075843702,200.70865654923,215.573593133701));
#17763=CARTESIAN_POINT('',(19.2205075843702,200.70865654923,211.073593133701));
#17764=CARTESIAN_POINT('Origin',(36.6954328642313,102.247359653123,215.573593133701));
#17765=CARTESIAN_POINT('Origin',(36.6954328642313,102.247359653123,215.573593133701));
#17766=CARTESIAN_POINT('',(68.8536755000203,196.935518525169,215.573593133701));
#17767=CARTESIAN_POINT('Origin',(36.6954328642313,102.247359653123,215.573593133701));
#17768=CARTESIAN_POINT('',(68.8536755000203,196.935518525169,211.073593133701));
#17769=CARTESIAN_POINT('',(68.8536755000203,196.935518525169,211.073593133701));
#17770=CARTESIAN_POINT('',(24.6736703960697,201.522115896385,211.073593133701));
#17771=CARTESIAN_POINT('Origin',(36.6954328642313,102.247359653123,211.073593133701));
#17772=CARTESIAN_POINT('Ctrl Pts',(24.6736703960694,201.522115896385,211.073593133701));
#17773=CARTESIAN_POINT('Ctrl Pts',(21.5391004439812,201.142532437006,211.073593133701));
#17774=CARTESIAN_POINT('Ctrl Pts',(18.1382702274613,200.570522874585,210.784723883084));
#17775=CARTESIAN_POINT('Ctrl Pts',(14.7712835464547,199.814423097892,210.39380950634));
#17776=CARTESIAN_POINT('Ctrl Pts',(14.7577154236595,199.811373238515,210.392231751654));
#17777=CARTESIAN_POINT('Ctrl Pts',(14.7441480327787,199.808320566023,210.390652633755));
#17778=CARTESIAN_POINT('Origin',(-292.116850606278,98.3518483080855,253.073593133701));
#17779=CARTESIAN_POINT('',(10.5134668616108,198.923857134272,206.096933730814));
#17780=CARTESIAN_POINT('',(13.3382261621522,199.862598895781,209.073593133701));
#17781=CARTESIAN_POINT('',(-118.511980891635,156.045309542559,70.1332032307269));
#17782=CARTESIAN_POINT('',(-253.322233103775,111.244319381425,209.073593133701));
#17783=CARTESIAN_POINT('',(-292.116850606278,98.3518483080855,209.073593133701));
#17784=CARTESIAN_POINT('',(-250.497473803234,112.183061142934,206.096933730814));
#17785=CARTESIAN_POINT('',(-293.596873185455,97.8599979041293,251.513983036674));
#17786=CARTESIAN_POINT('',(-214.933263098157,124.001983129515,190.573593133701));
#17787=CARTESIAN_POINT('Origin',(-214.933263098157,124.001983129515,243.573593133701));
#17788=CARTESIAN_POINT('',(-25.0507438434661,187.104935147691,190.573593133701));
#17789=CARTESIAN_POINT('',(-292.116850606278,98.3518483080855,190.573593133701));
#17790=CARTESIAN_POINT('Origin',(-25.0507438434661,187.104935147691,243.573593133701));
#17791=CARTESIAN_POINT('Origin',(-293.958747352154,37.7397376070391,211.073593133701));
#17792=CARTESIAN_POINT('',(264.041252647846,37.7397376070391,215.573593133701));
#17793=CARTESIAN_POINT('',(287.041252647846,37.7397376070391,215.573593133701));
#17794=CARTESIAN_POINT('',(-293.958747352154,37.7397376070391,215.573593133701));
#17795=CARTESIAN_POINT('',(264.041252647846,37.7397376070391,211.073593133701));
#17796=CARTESIAN_POINT('',(264.041252647846,37.7397376070391,211.073593133701));
#17797=CARTESIAN_POINT('',(287.041252647846,37.7397376070391,211.073593133701));
#17798=CARTESIAN_POINT('',(-293.958747352154,37.7397376070391,211.073593133701));
#17799=CARTESIAN_POINT('',(287.041252647846,37.7397376070391,211.073593133701));
#17800=CARTESIAN_POINT('Origin',(-293.959747352154,79.7397376070391,137.073593133701));
#17801=CARTESIAN_POINT('',(176.041252647846,62.8635864382735,193.919576017964));
#17802=CARTESIAN_POINT('',(176.041252647846,79.7397376070391,137.073593133701));
#17803=CARTESIAN_POINT('',(173.041252647846,62.8635864382735,193.919576017964));
#17804=CARTESIAN_POINT('',(-293.959747352154,62.8635864382735,193.919576017964));
#17805=CARTESIAN_POINT('',(173.041252647846,79.7397376070394,137.0735931337));
#17806=CARTESIAN_POINT('',(236.80135487697,62.8635864382735,193.919576017964));
#17807=CARTESIAN_POINT('',(221.30495438235,98.0959760916413,75.2420529750407));
#17808=CARTESIAN_POINT('',(233.775887951372,62.8635864382735,193.919576017964));
#17809=CARTESIAN_POINT('',(-293.959747352154,62.8635864382735,193.919576017964));
#17810=CARTESIAN_POINT('',(218.326162231598,97.9898570057988,75.5995067378785));
#17811=CARTESIAN_POINT('Origin',(-293.959747352154,53.2771177754925,191.073593133701));
#17812=CARTESIAN_POINT('',(176.041252647846,53.2771177754925,201.073593133701));
#17813=CARTESIAN_POINT('Origin',(176.041252647846,53.2771177754925,191.073593133701));
#17814=CARTESIAN_POINT('',(173.041252647846,53.2771177754925,201.073593133701));
#17815=CARTESIAN_POINT('',(-293.959747352154,53.2771177754925,201.073593133701));
#17816=CARTESIAN_POINT('Origin',(173.041252647846,53.2771177754925,191.073593133701));
#17817=CARTESIAN_POINT('Origin',(-293.959747352154,53.2771177754925,191.073593133701));
#17818=CARTESIAN_POINT('',(234.71002873497,53.2771177754925,201.073593133701));
#17819=CARTESIAN_POINT('',(237.735495660568,53.2771177754925,201.073593133701));
#17820=CARTESIAN_POINT('',(-293.959747352154,53.2771177754925,201.073593133701));
#17821=CARTESIAN_POINT('Origin',(233.404271747693,53.277117775496,191.073593133705));
#17822=CARTESIAN_POINT('Origin',(236.42973867329,53.2771177754941,191.073593133703));
#17823=CARTESIAN_POINT('Origin',(-293.959747352154,53.2771177754925,201.073593133701));
#17824=CARTESIAN_POINT('',(176.041252647846,39.7397376070391,201.073593133701));
#17825=CARTESIAN_POINT('',(176.041252647846,53.2771177754925,201.073593133701));
#17826=CARTESIAN_POINT('',(173.041252647846,39.7397376070391,201.073593133701));
#17827=CARTESIAN_POINT('',(-293.959747352154,39.7397376070391,201.073593133701));
#17828=CARTESIAN_POINT('',(173.041252647846,53.2771177754925,201.073593133701));
#17829=CARTESIAN_POINT('Origin',(-293.959747352154,53.2771177754925,201.073593133701));
#17830=CARTESIAN_POINT('',(237.735495660568,39.7397376070391,201.073593133701));
#17831=CARTESIAN_POINT('',(237.735495660568,53.2771177754925,201.073593133701));
#17832=CARTESIAN_POINT('',(234.71002873497,39.7397376070391,201.073593133701));
#17833=CARTESIAN_POINT('',(-293.959747352154,39.7397376070391,201.073593133701));
#17834=CARTESIAN_POINT('',(234.71002873497,53.2771177754925,201.073593133701));
#17835=CARTESIAN_POINT('Origin',(173.041252647846,88.7397376070391,167.073593133701));
#17836=CARTESIAN_POINT('',(173.041252647846,82.7397376070391,211.073593133701));
#17837=CARTESIAN_POINT('',(173.041252647846,88.7397376070391,211.073593133701));
#17838=CARTESIAN_POINT('',(173.041252647846,82.7397376070391,167.073593133701));
#17839=CARTESIAN_POINT('Origin',(173.041252647846,39.7397376070391,203.073593133701));
#17840=CARTESIAN_POINT('Origin',(239.041252647847,88.7397376070391,211.073593133701));
#17841=CARTESIAN_POINT('',(239.041252647847,82.7397376070391,211.073593133701));
#17842=CARTESIAN_POINT('',(239.041252647847,82.7397376070391,211.073593133701));
#17843=CARTESIAN_POINT('',(239.041252647847,88.7397376070391,211.073593133701));
#17844=CARTESIAN_POINT('Origin',(237.996647058024,39.7397376070393,203.073593133701));
#17845=CARTESIAN_POINT('Origin',(-276.958747352154,52.7397376070391,211.073593133701));
#17846=CARTESIAN_POINT('',(262.309201840278,36.7397376070391,211.073593133701));
#17847=CARTESIAN_POINT('Origin',(264.041252647846,35.7397376070391,211.073593133701));
#17848=CARTESIAN_POINT('',(81.7733034554153,36.7397376070391,211.073593133701));
#17849=CARTESIAN_POINT('',(-276.958747352154,36.7397376070391,211.073593133701));
#17850=CARTESIAN_POINT('Origin',(80.0412526478464,35.7397376070391,211.073593133701));
#17851=CARTESIAN_POINT('',(-293.958747352154,52.7397376070391,211.073593133701));
#17852=CARTESIAN_POINT('Origin',(-278.958747352154,52.7397376070391,211.073593133701));
#17853=CARTESIAN_POINT('',(-293.958747352154,86.9180139243132,211.073593133701));
#17854=CARTESIAN_POINT('',(-293.958747352154,97.7397376070391,211.073593133701));
#17855=CARTESIAN_POINT('',(-283.689260493489,101.152558013242,211.073593133701));
#17856=CARTESIAN_POINT('Origin',(-278.958747352154,86.9180139243132,211.073593133701));
#17857=CARTESIAN_POINT('',(37.0412526478464,207.739737607039,211.073593133701));
#17858=CARTESIAN_POINT('',(-254.589437230121,108.715645084056,211.073593133701));
#17859=CARTESIAN_POINT('',(-256.639326258033,114.883947522592,211.073593133701));
#17860=CARTESIAN_POINT('',(-291.486115520766,96.4539090962283,211.073593133701));
#17861=CARTESIAN_POINT('',(291.864989043215,121.19582713314,211.073593133701));
#17862=CARTESIAN_POINT('',(302.041252647846,117.739737607039,211.073593133701));
#17863=CARTESIAN_POINT('',(302.041252647846,106.992603302334,211.073593133701));
#17864=CARTESIAN_POINT('Origin',(287.041252647846,106.992603302334,211.073593133701));
#17865=CARTESIAN_POINT('',(302.041252647846,52.7397376070391,211.073593133701));
#17866=CARTESIAN_POINT('',(302.041252647846,37.7397376070391,211.073593133701));
#17867=CARTESIAN_POINT('Origin',(287.041252647846,52.7397376070391,211.073593133701));
#17868=CARTESIAN_POINT('',(179.041252647847,88.7397376070391,211.073593133701));
#17869=CARTESIAN_POINT('',(232.990318796651,88.7397376070391,211.073593133701));
#17870=CARTESIAN_POINT('',(173.041252647846,88.7397376070391,211.073593133701));
#17871=CARTESIAN_POINT('Origin',(179.041252647847,82.7397376070391,211.073593133701));
#17872=CARTESIAN_POINT('',(82.0412526478464,37.7397376070391,211.073593133701));
#17873=CARTESIAN_POINT('Origin',(232.990318796656,82.7397376070436,211.073593133701));
#17874=CARTESIAN_POINT('Origin',(-276.958747352154,52.7397376070391,290.573593133701));
#17875=CARTESIAN_POINT('',(264.041252647846,37.7397376070391,290.573593133701));
#17876=CARTESIAN_POINT('',(287.041252647846,37.7397376070391,290.573593133701));
#17877=CARTESIAN_POINT('',(-293.958747352154,37.7397376070391,290.573593133701));
#17878=CARTESIAN_POINT('',(262.309201840278,36.7397376070391,290.573593133701));
#17879=CARTESIAN_POINT('Origin',(264.041252647846,35.7397376070391,290.573593133701));
#17880=CARTESIAN_POINT('',(81.7733034554153,36.7397376070391,290.573593133701));
#17881=CARTESIAN_POINT('',(-276.958747352154,36.7397376070391,290.573593133701));
#17882=CARTESIAN_POINT('Origin',(80.0412526478464,35.7397376070391,290.573593133701));
#17883=CARTESIAN_POINT('',(-293.958747352154,52.7397376070391,290.573593133701));
#17884=CARTESIAN_POINT('Origin',(-278.958747352154,52.7397376070391,290.573593133701));
#17885=CARTESIAN_POINT('',(-293.958747352154,86.9180139243132,290.573593133701));
#17886=CARTESIAN_POINT('',(-293.958747352154,97.7397376070391,290.573593133701));
#17887=CARTESIAN_POINT('',(-283.689260493489,101.152558013242,290.573593133701));
#17888=CARTESIAN_POINT('Origin',(-278.958747352154,86.9180139243132,290.573593133701));
#17889=CARTESIAN_POINT('',(-259.490535542311,109.194430353513,290.573593133701));
#17890=CARTESIAN_POINT('',(37.0412526478464,207.739737607039,290.573593133701));
#17891=CARTESIAN_POINT('',(-257.691868353317,110.319062001314,290.573593133701));
#17892=CARTESIAN_POINT('Origin',(-260.909689484712,113.464793580191,290.573593133701));
#17893=CARTESIAN_POINT('',(16.0838694668338,201.301935597134,290.573593133701));
#17894=CARTESIAN_POINT('',(15.0784816026316,200.967818784257,290.573593133701));
#17895=CARTESIAN_POINT('',(19.2205075843702,200.70865654923,290.573593133701));
#17896=CARTESIAN_POINT('Origin',(18.4341359467765,205.139414909555,290.573593133701));
#17897=CARTESIAN_POINT('Origin',(36.6954328642313,102.247359653123,290.573593133701));
#17898=CARTESIAN_POINT('',(68.8536755000203,196.935518525169,290.573593133701));
#17899=CARTESIAN_POINT('Origin',(36.6954328642313,102.247359653123,290.573593133701));
#17900=CARTESIAN_POINT('',(291.864989043215,121.19582713314,290.573593133701));
#17901=CARTESIAN_POINT('',(302.041252647846,117.739737607039,290.573593133701));
#17902=CARTESIAN_POINT('',(302.041252647846,106.992603302334,290.573593133701));
#17903=CARTESIAN_POINT('Origin',(287.041252647846,106.992603302334,290.573593133701));
#17904=CARTESIAN_POINT('',(302.041252647846,52.7397376070391,290.573593133701));
#17905=CARTESIAN_POINT('',(302.041252647846,37.7397376070391,290.573593133701));
#17906=CARTESIAN_POINT('Origin',(287.041252647846,52.7397376070391,290.573593133701));
#17907=CARTESIAN_POINT('Origin',(37.0412526478464,207.739737607039,295.073593133701));
#17908=CARTESIAN_POINT('',(-259.490535542311,109.194430353513,295.073593133701));
#17909=CARTESIAN_POINT('',(-283.689260493489,101.152558013242,295.073593133701));
#17910=CARTESIAN_POINT('',(37.0412526478464,207.739737607039,295.073593133701));
#17911=CARTESIAN_POINT('',(-259.490535542311,109.194430353513,290.573593133701));
#17912=CARTESIAN_POINT('',(-283.689260493489,101.152558013242,295.073593133701));
#17913=CARTESIAN_POINT('Origin',(-293.959747352154,53.2771177754925,305.073593133701));
#17914=CARTESIAN_POINT('',(173.041252647846,39.7397376070391,305.073593133701));
#17915=CARTESIAN_POINT('',(173.041252647846,53.2771177754925,305.073593133701));
#17916=CARTESIAN_POINT('',(173.041252647846,53.2771177754925,305.073593133701));
#17917=CARTESIAN_POINT('',(176.041252647846,39.7397376070391,305.073593133701));
#17918=CARTESIAN_POINT('',(-293.959747352154,39.7397376070391,305.073593133701));
#17919=CARTESIAN_POINT('',(176.041252647846,53.2771177754925,305.073593133701));
#17920=CARTESIAN_POINT('',(176.041252647846,53.2771177754925,305.073593133701));
#17921=CARTESIAN_POINT('',(-293.959747352154,53.2771177754925,305.073593133701));
#17922=CARTESIAN_POINT('Origin',(-293.959747352154,53.2771177754925,315.073593133701));
#17923=CARTESIAN_POINT('',(176.041252647846,62.8635864382735,312.227610249438));
#17924=CARTESIAN_POINT('Origin',(176.041252647846,53.2771177754925,315.073593133701));
#17925=CARTESIAN_POINT('',(173.041252647846,62.8635864382735,312.227610249438));
#17926=CARTESIAN_POINT('',(-293.959747352154,62.8635864382735,312.227610249438));
#17927=CARTESIAN_POINT('Origin',(173.041252647846,53.2771177754925,315.073593133701));
#17928=CARTESIAN_POINT('Origin',(-276.958747352154,52.7397376070391,295.073593133701));
#17929=CARTESIAN_POINT('',(81.7733034554153,36.7397376070391,295.073593133701));
#17930=CARTESIAN_POINT('Origin',(80.0412526478464,35.7397376070391,295.073593133701));
#17931=CARTESIAN_POINT('',(262.309201840278,36.7397376070391,295.073593133701));
#17932=CARTESIAN_POINT('',(-276.958747352154,36.7397376070391,295.073593133701));
#17933=CARTESIAN_POINT('',(264.041252647846,37.7397376070391,295.073593133701));
#17934=CARTESIAN_POINT('Origin',(264.041252647846,35.7397376070391,295.073593133701));
#17935=CARTESIAN_POINT('',(287.041252647846,37.7397376070391,295.073593133701));
#17936=CARTESIAN_POINT('',(-293.958747352154,37.7397376070391,295.073593133701));
#17937=CARTESIAN_POINT('',(302.041252647846,52.7397376070391,295.073593133701));
#17938=CARTESIAN_POINT('Origin',(287.041252647846,52.7397376070391,295.073593133701));
#17939=CARTESIAN_POINT('',(302.041252647846,106.992603302334,295.073593133701));
#17940=CARTESIAN_POINT('',(302.041252647846,37.7397376070391,295.073593133701));
#17941=CARTESIAN_POINT('',(291.864989043215,121.19582713314,295.073593133701));
#17942=CARTESIAN_POINT('Origin',(287.041252647846,106.992603302334,295.073593133701));
#17943=CARTESIAN_POINT('',(68.8536755000203,196.935518525169,295.073593133701));
#17944=CARTESIAN_POINT('',(302.041252647846,117.739737607039,295.073593133701));
#17945=CARTESIAN_POINT('',(24.6736703960697,201.522115896385,295.073593133701));
#17946=CARTESIAN_POINT('Origin',(36.6954328642313,102.247359653123,295.073593133701));
#17947=CARTESIAN_POINT('',(-254.589437230121,108.715645084056,295.073593133701));
#17948=CARTESIAN_POINT('',(-291.486115520766,96.4539090962283,295.073593133701));
#17949=CARTESIAN_POINT('',(-256.639326258033,114.883947522592,295.073593133701));
#17950=CARTESIAN_POINT('',(-240.062069061508,65.0014735948669,295.073593133701));
#17951=CARTESIAN_POINT('Origin',(-260.909689484712,113.464793580191,295.073593133701));
#17952=CARTESIAN_POINT('',(-293.958747352154,86.9180139243132,295.073593133701));
#17953=CARTESIAN_POINT('Origin',(-278.958747352154,86.9180139243132,295.073593133701));
#17954=CARTESIAN_POINT('',(-293.958747352154,52.7397376070391,295.073593133701));
#17955=CARTESIAN_POINT('',(-293.958747352154,97.7397376070391,295.073593133701));
#17956=CARTESIAN_POINT('Origin',(-278.958747352154,52.7397376070391,295.073593133701));
#17957=CARTESIAN_POINT('',(173.041252647846,82.7397376070391,295.073593133701));
#17958=CARTESIAN_POINT('',(173.041252647846,88.7397376070391,295.073593133701));
#17959=CARTESIAN_POINT('',(179.041252647847,88.7397376070391,295.073593133701));
#17960=CARTESIAN_POINT('Origin',(179.041252647847,82.7397376070391,295.073593133701));
#17961=CARTESIAN_POINT('',(232.990318796651,88.7397376070391,295.073593133701));
#17962=CARTESIAN_POINT('',(173.041252647846,88.7397376070391,295.073593133701));
#17963=CARTESIAN_POINT('',(239.041252647847,82.7397376070391,295.073593133701));
#17964=CARTESIAN_POINT('Origin',(232.990318796658,82.7397376070451,295.073593133701));
#17965=CARTESIAN_POINT('',(239.041252647847,88.7397376070391,295.073593133701));
#17966=CARTESIAN_POINT('',(82.0412526478464,37.7397376070391,295.073593133701));
#17967=CARTESIAN_POINT('Origin',(-293.958747352154,97.7397376070391,295.073593133701));
#17968=CARTESIAN_POINT('',(-293.958747352154,52.7397376070391,295.073593133701));
#17969=CARTESIAN_POINT('',(-293.958747352154,86.9180139243132,295.073593133701));
#17970=CARTESIAN_POINT('Origin',(-293.958747352154,37.7397376070391,295.073593133701));
#17971=CARTESIAN_POINT('',(264.041252647846,37.7397376070391,295.073593133701));
#17972=CARTESIAN_POINT('',(287.041252647846,37.7397376070391,295.073593133701));
#17973=CARTESIAN_POINT('Origin',(302.041252647846,37.7397376070391,295.073593133701));
#17974=CARTESIAN_POINT('',(302.041252647846,52.7397376070391,295.073593133701));
#17975=CARTESIAN_POINT('',(302.041252647846,106.992603302334,295.073593133701));
#17976=CARTESIAN_POINT('Origin',(302.041252647846,117.739737607039,295.073593133701));
#17977=CARTESIAN_POINT('',(291.864989043215,121.19582713314,295.073593133701));
#17978=CARTESIAN_POINT('',(68.8536755000203,196.935518525169,295.073593133701));
#17979=CARTESIAN_POINT('Origin',(-276.958747352154,52.7397376070391,307.323593133701));
#17980=CARTESIAN_POINT('Origin',(173.041252647846,88.7397376070391,339.073593133701));
#17981=CARTESIAN_POINT('',(173.041252647846,82.7397376070391,339.073593133701));
#17982=CARTESIAN_POINT('',(173.041252647846,70.8334876070391,339.073593133701));
#17983=CARTESIAN_POINT('',(173.041252647846,88.7397376070391,339.073593133701));
#17984=CARTESIAN_POINT('',(173.041252647846,82.7397376070391,295.073593133701));
#17985=CARTESIAN_POINT('Origin',(173.041252647846,39.7397376070391,303.073593133701));
#17986=CARTESIAN_POINT('',(173.041252647846,79.7397376070394,369.073593133702));
#17987=CARTESIAN_POINT('Origin',(203.041252647846,88.7397376070391,339.073593133701));
#17988=CARTESIAN_POINT('',(232.788727075195,82.7397376070391,342.95789039244));
#17989=CARTESIAN_POINT('',(232.788727075195,71.9866383557274,342.95789039244));
#17990=CARTESIAN_POINT('',(232.788727075195,88.7397376070391,342.95789039244));
#17991=CARTESIAN_POINT('Origin',(203.041252647846,82.7397376070391,339.073593133701));
#17992=CARTESIAN_POINT('Origin',(203.041252647846,70.8334876070392,339.073593133701));
#17993=CARTESIAN_POINT('Origin',(239.041252647847,88.7397376070391,295.073593133701));
#17994=CARTESIAN_POINT('',(232.788727075195,82.7397376070391,342.95789039244));
#17995=CARTESIAN_POINT('',(236.80135487697,62.8635864382735,312.227610249438));
#17996=CARTESIAN_POINT('',(221.30495438235,98.0959760916413,430.905133292361));
#17997=CARTESIAN_POINT('',(237.735495660568,53.2771177754925,305.073593133701));
#17998=CARTESIAN_POINT('Origin',(236.42973867329,53.2771177754957,315.073593133697));
#17999=CARTESIAN_POINT('',(237.735495660568,39.7397376070391,305.073593133701));
#18000=CARTESIAN_POINT('',(237.735495660568,53.2771177754925,305.073593133701));
#18001=CARTESIAN_POINT('Origin',(237.996647058023,39.7397376070351,303.073593133704));
#18002=CARTESIAN_POINT('Origin',(203.041252647846,88.7397376070391,339.073593133701));
#18003=CARTESIAN_POINT('',(179.041252647846,88.7397376070391,339.073593133701));
#18004=CARTESIAN_POINT('',(226.839232189725,88.7397376070391,342.181030940692));
#18005=CARTESIAN_POINT('Origin',(203.041252647846,88.7397376070391,339.073593133701));
#18006=CARTESIAN_POINT('',(233.091757762377,88.7397376070391,294.296733681953));
#18007=CARTESIAN_POINT('',(179.041252647846,88.7397376070391,339.073593133701));
#18008=CARTESIAN_POINT('Origin',(-293.959747352154,53.2771177754925,305.073593133701));
#18009=CARTESIAN_POINT('',(234.71002873497,53.2771177754925,305.073593133701));
#18010=CARTESIAN_POINT('',(234.71002873497,39.7397376070391,305.073593133701));
#18011=CARTESIAN_POINT('',(234.71002873497,53.2771177754925,305.073593133701));
#18012=CARTESIAN_POINT('',(-293.959747352154,39.7397376070391,305.073593133701));
#18013=CARTESIAN_POINT('',(-293.959747352154,53.2771177754925,305.073593133701));
#18014=CARTESIAN_POINT('Origin',(-293.959747352154,53.2771177754925,315.073593133701));
#18015=CARTESIAN_POINT('',(233.775887951372,62.8635864382735,312.227610249438));
#18016=CARTESIAN_POINT('',(-293.959747352154,62.8635864382735,312.227610249438));
#18017=CARTESIAN_POINT('Origin',(233.404271747692,53.2771177754959,315.073593133697));
#18018=CARTESIAN_POINT('Origin',(-293.959747352154,79.7397376070391,369.073593133701));
#18019=CARTESIAN_POINT('',(176.041252647846,70.8334876070391,339.073593133701));
#18020=CARTESIAN_POINT('',(176.041252647846,79.7397376070391,369.073593133701));
#18021=CARTESIAN_POINT('',(229.81397963246,71.8713232808586,342.569460666566));
#18022=CARTESIAN_POINT('Origin',(203.041252647846,70.8334876070391,339.073593133701));
#18023=CARTESIAN_POINT('',(218.326162231599,97.9898570057982,430.547679529521));
#18024=CARTESIAN_POINT('Origin',(203.041252647846,85.7397376070391,339.073593133701));
#18025=CARTESIAN_POINT('',(231.506382410955,85.7397376070391,298.714756191828));
#18026=CARTESIAN_POINT('',(225.847649708814,85.7397376070391,342.051554365401));
#18027=CARTESIAN_POINT('',(225.847649708814,85.7397376070391,342.051554365401));
#18028=CARTESIAN_POINT('',(180.041252647846,85.7397376070391,339.073593133701));
#18029=CARTESIAN_POINT('Origin',(203.041252647846,85.7397376070391,339.073593133701));
#18030=CARTESIAN_POINT('',(180.041252647846,85.7397376070391,299.047792462302));
#18031=CARTESIAN_POINT('',(180.041252647846,85.7397376070391,339.073593133701));
#18032=CARTESIAN_POINT('',(202.781289236061,85.7397376070391,298.900639292561));
#18033=CARTESIAN_POINT('Origin',(176.041252647846,182.009983898606,305.073593133701));
#18034=CARTESIAN_POINT('Origin',(176.041252647846,39.7397376070391,303.073593133701));
#18035=CARTESIAN_POINT('',(176.041252647846,81.7397376070391,299.047792462302));
#18036=CARTESIAN_POINT('',(176.041252647846,85.7397376070391,299.047792462302));
#18037=CARTESIAN_POINT('',(176.041252647846,81.7397376070391,339.073593133701));
#18038=CARTESIAN_POINT('',(176.041252647846,81.7397376070391,305.073593133701));
#18039=CARTESIAN_POINT('',(176.041252647846,182.009983898606,339.073593133701));
#18040=CARTESIAN_POINT('Origin',(203.041252647846,182.009983898606,339.073593133701));
#18041=CARTESIAN_POINT('',(229.81397963246,81.7397376070391,342.569460666566));
#18042=CARTESIAN_POINT('Origin',(203.041252647846,81.7397376070391,339.073593133701));
#18043=CARTESIAN_POINT('',(229.81397963246,182.009983898606,342.569460666566));
#18044=CARTESIAN_POINT('Origin',(233.826607434235,182.009983898606,311.839180523564));
#18045=CARTESIAN_POINT('Origin',(234.971180132426,39.7397376070352,303.073593133704));
#18046=CARTESIAN_POINT('',(235.472712334602,81.7397376070391,299.232662492993));
#18047=CARTESIAN_POINT('',(233.826607434235,81.7397376070391,311.839180523564));
#18048=CARTESIAN_POINT('',(235.472712334602,37.7397376070391,299.232662492993));
#18049=CARTESIAN_POINT('Origin',(176.041252647846,182.009983898606,295.073593133701));
#18050=CARTESIAN_POINT('',(180.015368768859,37.7397376070391,295.047876210078));
#18051=CARTESIAN_POINT('',(231.480498531968,37.7397376070391,294.714839939603));
#18052=CARTESIAN_POINT('',(176.041252647846,37.7397376070391,295.073593133701));
#18053=CARTESIAN_POINT('',(231.480498531968,81.7397376070391,294.714839939603));
#18054=CARTESIAN_POINT('',(231.480498531968,85.7397376070391,294.714839939603));
#18055=CARTESIAN_POINT('',(180.015368768859,81.7397376070391,295.047876210078));
#18056=CARTESIAN_POINT('',(176.041252647846,81.7397376070391,295.073593133701));
#18057=CARTESIAN_POINT('',(180.015368768859,37.7397376070391,295.047876210078));
#18058=CARTESIAN_POINT('Origin',(36.6954328642313,102.247359653123,295.073593133701));
#18059=CARTESIAN_POINT('',(19.2205075843702,200.70865654923,291.2246677273));
#18060=CARTESIAN_POINT('',(19.2205075843702,200.70865654923,295.073593133701));
#18061=CARTESIAN_POINT('',(14.7441480327787,199.808320566024,295.756533633647));
#18062=CARTESIAN_POINT('Origin',(36.6954313613018,102.247367094447,305.692991109406));
#18063=CARTESIAN_POINT('Ctrl Pts',(14.7441480327787,199.808320566023,295.756533633647));
#18064=CARTESIAN_POINT('Ctrl Pts',(14.7577154236595,199.811373238515,295.754954515747));
#18065=CARTESIAN_POINT('Ctrl Pts',(14.7712835464547,199.814423097892,295.753376761062));
#18066=CARTESIAN_POINT('Ctrl Pts',(18.1382702274613,200.570522874585,295.362462384317));
#18067=CARTESIAN_POINT('Ctrl Pts',(21.5391004439812,201.142532437006,295.073593133701));
#18068=CARTESIAN_POINT('Ctrl Pts',(24.6736703960694,201.522115896385,295.073593133701));
#18069=CARTESIAN_POINT('Origin',(36.6954328642313,102.247359653123,290.573593133701));
#18070=CARTESIAN_POINT('Origin',(287.041252647846,52.7397376070391,295.073593133701));
#18071=CARTESIAN_POINT('Origin',(287.041252647846,106.992603302334,295.073593133701));
#18072=CARTESIAN_POINT('Origin',(-278.958747352154,52.7397376070391,295.073593133701));
#18073=CARTESIAN_POINT('Origin',(-278.958747352154,86.9180139243132,295.073593133701));
#18074=CARTESIAN_POINT('Origin',(-293.536004548678,102.622211534764,315.573593133701));
#18075=CARTESIAN_POINT('',(-216.352417040558,128.272346356194,315.573593133701));
#18076=CARTESIAN_POINT('',(-26.4698977858668,191.375298374369,315.573593133701));
#18077=CARTESIAN_POINT('',(-293.536004548678,102.622211534764,315.573593133701));
#18078=CARTESIAN_POINT('',(-214.933263098157,124.001983129515,315.573593133701));
#18079=CARTESIAN_POINT('',(-216.352417040558,128.272346356194,315.573593133701));
#18080=CARTESIAN_POINT('',(-25.0507438434661,187.104935147691,315.573593133701));
#18081=CARTESIAN_POINT('',(-292.116850606278,98.3518483080855,315.573593133701));
#18082=CARTESIAN_POINT('',(-26.4698977858668,191.375298374369,315.573593133701));
#18083=CARTESIAN_POINT('Origin',(-292.116850606278,98.3518483080855,253.073593133701));
#18084=CARTESIAN_POINT('',(-253.322233103775,111.244319381425,297.073593133701));
#18085=CARTESIAN_POINT('',(-250.497473803234,112.183061142934,300.050252536588));
#18086=CARTESIAN_POINT('',(-293.596873185455,97.8599979041293,254.633203230727));
#18087=CARTESIAN_POINT('',(13.3382261621522,199.862598895781,297.073593133701));
#18088=CARTESIAN_POINT('',(-292.116850606278,98.3518483080855,297.073593133701));
#18089=CARTESIAN_POINT('',(10.5134668616108,198.923857134272,300.050252536588));
#18090=CARTESIAN_POINT('',(-118.511980891635,156.045309542559,436.013983036675));
#18091=CARTESIAN_POINT('Origin',(-25.050743843466,187.104935147691,262.573593133701));
#18092=CARTESIAN_POINT('Origin',(-214.933263098157,124.001983129515,262.573593133701));
#18093=CARTESIAN_POINT('Origin',(-295.016027127856,102.130361130808,254.633203230727));
#18094=CARTESIAN_POINT('',(-251.916627745634,116.453424369613,300.050252536588));
#18095=CARTESIAN_POINT('',(-295.016027127856,102.130361130808,254.633203230727));
#18096=CARTESIAN_POINT('Origin',(-252.691498018264,109.346380169568,297.0735931337));
#18097=CARTESIAN_POINT('',(-251.916627745634,116.453424369613,300.050252536588));
#18098=CARTESIAN_POINT('Origin',(13.8170114316087,204.763697207971,253.073593133701));
#18099=CARTESIAN_POINT('',(13.8170114316087,204.763697207971,295.073593133701));
#18100=CARTESIAN_POINT('',(14.1637727200978,203.720260967154,295.073593133701));
#18101=CARTESIAN_POINT('',(13.8170114316087,204.763697207971,295.073593133701));
#18102=CARTESIAN_POINT('',(14.1637727200979,203.720260967154,291.819075083293));
#18103=CARTESIAN_POINT('',(14.1637727200979,203.720260967154,253.073593133701));
#18104=CARTESIAN_POINT('',(13.8170114316087,204.763697207971,294.573593133701));
#18105=CARTESIAN_POINT('Origin',(15.0784816026316,200.967818784257,294.573593133701));
#18106=CARTESIAN_POINT('',(13.8170114316087,204.763697207971,253.073593133701));
#18107=CARTESIAN_POINT('Origin',(-119.931134834035,160.315672769238,436.013983036675));
#18108=CARTESIAN_POINT('',(9.09431291921015,203.194220360951,300.050252536588));
#18109=CARTESIAN_POINT('',(-119.931134834035,160.315672769238,436.013983036675));
#18110=CARTESIAN_POINT('',(9.09431291921009,203.194220360951,300.050252536588));
#18111=CARTESIAN_POINT('Origin',(13.9689612476602,197.964659683904,297.073593133711));
#18112=CARTESIAN_POINT('Origin',(18.434135946777,205.139414909556,290.5735931337));
#18113=CARTESIAN_POINT('Origin',(-293.536004548678,102.622211534764,253.073593133701));
#18114=CARTESIAN_POINT('',(-256.639326258033,114.883947522592,294.573593133701));
#18115=CARTESIAN_POINT('',(-256.639326258033,114.883947522592,294.573593133701));
#18116=CARTESIAN_POINT('',(-256.639326258033,114.883947522592,253.073593133701));
#18117=CARTESIAN_POINT('Origin',(-216.352417040558,128.272346356194,262.573593133701));
#18118=CARTESIAN_POINT('Origin',(-26.4698977858667,191.375298374369,262.573593133701));
#18119=CARTESIAN_POINT('Origin',(277.041252647846,78.7397376070391,283.573593133701));
#18120=CARTESIAN_POINT('Origin',(37.0412526478464,187.739737607039,273.573593133701));
#18121=CARTESIAN_POINT('Origin',(11.0412526478464,112.739737607039,285.573593133701));
#18122=CARTESIAN_POINT('Origin',(-293.958747352154,97.7397376070391,211.073593133701));
#18123=CARTESIAN_POINT('',(-293.958747352154,52.7397376070391,215.573593133701));
#18124=CARTESIAN_POINT('',(-293.958747352154,52.7397376070391,211.073593133701));
#18125=CARTESIAN_POINT('',(-293.958747352154,86.9180139243132,215.573593133701));
#18126=CARTESIAN_POINT('',(-293.958747352154,97.7397376070391,215.573593133701));
#18127=CARTESIAN_POINT('',(-293.958747352154,86.9180139243132,211.073593133701));
#18128=CARTESIAN_POINT('Origin',(37.0412526478464,207.739737607039,211.073593133701));
#18129=CARTESIAN_POINT('',(-283.689260493489,101.152558013242,215.573593133701));
#18130=CARTESIAN_POINT('',(37.0412526478464,207.739737607039,215.573593133701));
#18131=CARTESIAN_POINT('',(-283.689260493489,101.152558013242,211.073593133701));
#18132=CARTESIAN_POINT('Origin',(302.041252647846,117.739737607039,211.073593133701));
#18133=CARTESIAN_POINT('',(291.864989043215,121.19582713314,215.573593133701));
#18134=CARTESIAN_POINT('',(302.041252647846,117.739737607039,215.573593133701));
#18135=CARTESIAN_POINT('',(291.864989043215,121.19582713314,211.073593133701));
#18136=CARTESIAN_POINT('Origin',(302.041252647846,37.7397376070391,211.073593133701));
#18137=CARTESIAN_POINT('',(302.041252647846,52.7397376070391,215.573593133701));
#18138=CARTESIAN_POINT('',(302.041252647846,106.992603302334,215.573593133701));
#18139=CARTESIAN_POINT('',(302.041252647846,37.7397376070391,215.573593133701));
#18140=CARTESIAN_POINT('',(302.041252647846,52.7397376070391,211.073593133701));
#18141=CARTESIAN_POINT('',(302.041252647846,106.992603302334,211.073593133701));
#18142=CARTESIAN_POINT('Origin',(-276.958747352154,52.7397376070391,215.573593133701));
#18143=CARTESIAN_POINT('',(81.7733034554153,36.7397376070391,215.573593133701));
#18144=CARTESIAN_POINT('Origin',(80.0412526478464,35.7397376070391,215.573593133701));
#18145=CARTESIAN_POINT('',(262.309201840278,36.7397376070391,215.573593133701));
#18146=CARTESIAN_POINT('',(-276.958747352154,36.7397376070391,215.573593133701));
#18147=CARTESIAN_POINT('Origin',(264.041252647846,35.7397376070391,215.573593133701));
#18148=CARTESIAN_POINT('Origin',(287.041252647846,52.7397376070391,215.573593133701));
#18149=CARTESIAN_POINT('Origin',(287.041252647846,106.992603302334,215.573593133701));
#18150=CARTESIAN_POINT('',(16.0838694668338,201.301935597134,215.573593133701));
#18151=CARTESIAN_POINT('Origin',(18.4341359467765,205.139414909555,215.573593133701));
#18152=CARTESIAN_POINT('',(-255.37785608701,111.088069098878,215.573593133701));
#18153=CARTESIAN_POINT('Origin',(-278.958747352154,86.9180139243132,215.573593133701));
#18154=CARTESIAN_POINT('Origin',(-278.958747352154,52.7397376070391,215.573593133701));
#18155=CARTESIAN_POINT('Origin',(-276.958747352154,52.7397376070391,198.823593133701));
#18156=CARTESIAN_POINT('Origin',(203.041252647846,88.7397376070391,167.073593133701));
#18157=CARTESIAN_POINT('',(226.839232189725,88.7397376070391,163.966155326709));
#18158=CARTESIAN_POINT('',(179.041252647846,88.7397376070391,167.073593133701));
#18159=CARTESIAN_POINT('Origin',(176.041252647846,182.009983898606,211.073593133701));
#18160=CARTESIAN_POINT('',(180.041252647846,85.7397376070391,211.099477554629));
#18161=CARTESIAN_POINT('',(176.041252647846,85.7397376070391,211.073593133701));
#18162=CARTESIAN_POINT('',(180.015368768859,37.7397376070391,211.099310057324));
#18163=CARTESIAN_POINT('',(176.041252647846,37.7397376070391,211.073593133701));
#18164=CARTESIAN_POINT('',(180.015368768859,85.7396538592634,211.099310057324));
#18165=CARTESIAN_POINT('',(180.015368768859,85.7397376070391,211.099310057324));
#18166=CARTESIAN_POINT('Origin',(180.041272326363,81.733660909987,211.099477683049));
#18167=CARTESIAN_POINT('Origin',(176.041252647846,182.009983898606,167.073593133701));
#18168=CARTESIAN_POINT('Origin',(176.041252647846,39.7397376070391,203.073593133701));
#18169=CARTESIAN_POINT('',(176.041252647846,81.7397376070391,207.0993938051));
#18170=CARTESIAN_POINT('',(176.041252647846,81.7397376070391,211.073593133701));
#18171=CARTESIAN_POINT('',(176.041252647846,37.7397376070391,207.0993938051));
#18172=CARTESIAN_POINT('Origin',(234.760748217833,182.009983898606,201.462022859575));
#18173=CARTESIAN_POINT('Origin',(234.971180132426,39.7397376070408,203.073593133702));
#18174=CARTESIAN_POINT('',(229.81397963246,81.7397376070391,163.577725600835));
#18175=CARTESIAN_POINT('Origin',(203.041252647846,85.7397376070391,339.073593133701));
#18176=CARTESIAN_POINT('',(232.100175281465,85.7397376070391,211.97992916074));
#18177=CARTESIAN_POINT('',(180.041252647846,85.7397376070391,167.073593133701));
#18178=CARTESIAN_POINT('Origin',(287.041252647846,52.7397376070391,211.073593133701));
#18179=CARTESIAN_POINT('Origin',(287.041252647846,106.992603302334,211.073593133701));
#18180=CARTESIAN_POINT('Origin',(-278.958747352154,52.7397376070391,211.073593133701));
#18181=CARTESIAN_POINT('Origin',(-278.958747352154,86.9180139243132,211.073593133701));
#18182=CARTESIAN_POINT('Origin',(13.8170114316087,204.763697207971,253.073593133701));
#18183=CARTESIAN_POINT('',(13.8170114316087,204.763697207971,211.573593133701));
#18184=CARTESIAN_POINT('',(14.1637727200979,203.720260967154,214.328111184109));
#18185=CARTESIAN_POINT('Origin',(15.0784816026316,200.967818784257,211.573593133701));
#18186=CARTESIAN_POINT('',(14.1637727200978,203.720260967154,211.073593133701));
#18187=CARTESIAN_POINT('',(14.1637727200979,203.720260967154,211.073593133701));
#18188=CARTESIAN_POINT('',(13.8170114316087,204.763697207971,211.073593133701));
#18189=CARTESIAN_POINT('',(13.8170114316087,204.763697207971,211.073593133701));
#18190=CARTESIAN_POINT('',(13.8170114316087,204.763697207971,253.073593133701));
#18191=CARTESIAN_POINT('Origin',(-119.931134834035,160.315672769238,70.1332032307269));
#18192=CARTESIAN_POINT('',(9.09431291921009,203.194220360951,206.096933730814));
#18193=CARTESIAN_POINT('',(9.09431291921003,203.194220360951,206.096933730813));
#18194=CARTESIAN_POINT('',(-119.931134834035,160.315672769238,70.1332032307269));
#18195=CARTESIAN_POINT('Origin',(18.4341359467765,205.139414909555,215.573593133701));
#18196=CARTESIAN_POINT('Origin',(13.9689612476676,197.964659683866,209.073593133684));
#18197=CARTESIAN_POINT('Origin',(-293.536004548678,102.622211534764,190.573593133701));
#18198=CARTESIAN_POINT('',(-216.352417040558,128.272346356194,190.573593133701));
#18199=CARTESIAN_POINT('',(-216.352417040558,128.272346356194,190.573593133701));
#18200=CARTESIAN_POINT('',(-26.4698977858668,191.375298374369,190.573593133701));
#18201=CARTESIAN_POINT('',(-293.536004548678,102.622211534764,190.573593133701));
#18202=CARTESIAN_POINT('',(-26.4698977858668,191.375298374369,190.573593133701));
#18203=CARTESIAN_POINT('Origin',(-295.016027127856,102.130361130808,251.513983036674));
#18204=CARTESIAN_POINT('',(-251.916627745634,116.453424369613,206.096933730814));
#18205=CARTESIAN_POINT('',(-295.016027127856,102.130361130808,251.513983036674));
#18206=CARTESIAN_POINT('',(-251.916627745634,116.453424369613,206.096933730814));
#18207=CARTESIAN_POINT('Origin',(-252.691498018267,109.346380169569,209.073593133703));
#18208=CARTESIAN_POINT('Origin',(-293.536004548678,102.622211534764,253.073593133701));
#18209=CARTESIAN_POINT('',(13.8170114316088,204.763697207971,211.573593133701));
#18210=CARTESIAN_POINT('Origin',(-26.4698977858668,191.375298374369,243.573593133701));
#18211=CARTESIAN_POINT('Origin',(-216.352417040558,128.272346356194,243.573593133701));
#18212=CARTESIAN_POINT('Origin',(277.041252647846,78.7397376070391,222.573593133701));
#18213=CARTESIAN_POINT('Origin',(37.0412526478464,187.739737607039,232.573593133701));
#18214=CARTESIAN_POINT('Origin',(11.0412526478464,112.739737607039,220.573593133701));
#18215=CARTESIAN_POINT('Origin',(82.0412526478464,37.7397376070391,290.573593133701));
#18216=CARTESIAN_POINT('Origin',(231.506382410955,37.7397376070391,298.714756191828));
#18217=CARTESIAN_POINT('Origin',(180.041252647846,37.7397376070391,299.047792462302));
#18218=CARTESIAN_POINT('Origin',(82.0412526478464,34.7397376070391,290.573593133701));
#18219=CARTESIAN_POINT('',(262.041252647846,34.7397376070391,217.573593133701));
#18220=CARTESIAN_POINT('',(262.041252647846,34.7397376070391,288.573593133701));
#18221=CARTESIAN_POINT('',(262.041252647846,34.7397376070391,290.573593133701));
#18222=CARTESIAN_POINT('',(82.0412526478464,34.7397376070391,217.573593133701));
#18223=CARTESIAN_POINT('',(82.0412526478464,34.7397376070391,217.573593133701));
#18224=CARTESIAN_POINT('',(82.0412526478464,34.7397376070391,288.573593133701));
#18225=CARTESIAN_POINT('',(82.0412526478464,34.7397376070391,290.573593133701));
#18226=CARTESIAN_POINT('',(82.0412526478464,34.7397376070391,288.573593133701));
#18227=CARTESIAN_POINT('Origin',(82.0412526478464,37.7397376070391,215.573593133701));
#18228=CARTESIAN_POINT('Origin',(180.041252647846,37.7397376070391,207.0993938051));
#18229=CARTESIAN_POINT('Origin',(82.0412526478464,30.2397376070391,295.073593133701));
#18230=CARTESIAN_POINT('',(262.041252647846,30.2397376070391,288.573593133701));
#18231=CARTESIAN_POINT('',(262.041252647846,30.2397376070391,217.573593133701));
#18232=CARTESIAN_POINT('',(262.041252647846,30.2397376070391,295.073593133701));
#18233=CARTESIAN_POINT('',(82.0412526478464,30.2397376070391,288.573593133701));
#18234=CARTESIAN_POINT('',(82.0412526478464,30.2397376070391,288.573593133701));
#18235=CARTESIAN_POINT('',(82.0412526478464,30.2397376070391,217.573593133701));
#18236=CARTESIAN_POINT('',(82.0412526478464,30.2397376070391,295.073593133701));
#18237=CARTESIAN_POINT('',(82.0412526478464,30.2397376070391,217.573593133701));
#18238=CARTESIAN_POINT('Origin',(82.0412526478464,52.7397376070391,253.073593133701));
#18239=CARTESIAN_POINT('',(82.0412526478464,35.7397376070391,294.996209423033));
#18240=CARTESIAN_POINT('Origin',(82.0412526478464,36.7397376070391,288.573593133701));
#18241=CARTESIAN_POINT('',(82.0412526478464,35.7397376070391,290.30564394127));
#18242=CARTESIAN_POINT('',(82.0412526478464,35.7397376070391,290.573593133701));
#18243=CARTESIAN_POINT('Origin',(82.0412526478464,36.7397376070391,288.573593133701));
#18244=CARTESIAN_POINT('',(82.0412526478464,35.7397376070391,215.841542326132));
#18245=CARTESIAN_POINT('Origin',(82.0412526478464,36.7397376070391,217.573593133701));
#18246=CARTESIAN_POINT('',(82.0412526478464,35.7397376070391,211.150976844368));
#18247=CARTESIAN_POINT('',(82.0412526478464,35.7397376070391,253.073593133701));
#18248=CARTESIAN_POINT('Origin',(82.0412526478464,36.7397376070391,217.573593133701));
#18249=CARTESIAN_POINT('Origin',(262.041252647846,52.7397376070391,253.073593133701));
#18250=CARTESIAN_POINT('',(262.041252647846,35.7397376070391,290.30564394127));
#18251=CARTESIAN_POINT('',(262.041252647846,35.7397376070391,294.996209423033));
#18252=CARTESIAN_POINT('',(262.041252647846,35.7397376070391,253.073593133701));
#18253=CARTESIAN_POINT('Origin',(262.041252647846,36.7397376070391,288.573593133701));
#18254=CARTESIAN_POINT('',(262.041252647846,35.7397376070391,211.150976844368));
#18255=CARTESIAN_POINT('Origin',(262.041252647846,36.7397376070391,217.573593133701));
#18256=CARTESIAN_POINT('',(262.041252647846,35.7397376070391,215.841542326132));
#18257=CARTESIAN_POINT('',(262.041252647846,35.7397376070391,215.573593133701));
#18258=CARTESIAN_POINT('Origin',(262.041252647846,36.7397376070391,217.573593133701));
#18259=CARTESIAN_POINT('Origin',(262.041252647846,36.7397376070391,288.573593133701));
#18260=CARTESIAN_POINT('Origin',(-216.352417040558,128.272346356194,243.573593133701));
#18261=CARTESIAN_POINT('Origin',(-26.4698977858668,191.375298374369,243.573593133701));
#18262=CARTESIAN_POINT('Origin',(-216.352417040558,128.272346356194,262.573593133701));
#18263=CARTESIAN_POINT('Origin',(-26.4698977858667,191.375298374369,262.573593133701));
#18264=CARTESIAN_POINT('Origin',(180.041252647846,182.009983898606,207.0993938051));
#18265=CARTESIAN_POINT('Origin',(180.041252647849,81.7397376070372,207.099393805098));
#18266=CARTESIAN_POINT('Origin',(180.041252647846,81.7397376070391,339.073593133701));
#18267=CARTESIAN_POINT('Origin',(247.930162753351,81.7397376070391,333.212192331543));
#18268=CARTESIAN_POINT('Origin',(180.041252647846,182.009983898606,299.047792462302));
#18269=CARTESIAN_POINT('Origin',(180.041252647846,81.7397376070391,299.047792462302));
#18270=CARTESIAN_POINT('Origin',(231.506382410955,182.009983898606,298.714756191828));
#18271=CARTESIAN_POINT('Origin',(231.506382410955,81.7397376070391,298.714756191828));
#18272=CARTESIAN_POINT('Origin',(176.067136526834,81.7397376070391,299.073509385925));
#18273=CARTESIAN_POINT('Origin',(180.041252647846,81.7397376070391,299.047792462302));
#18274=CARTESIAN_POINT('Origin',(231.506382410955,81.7397376070391,298.714756191828));
#18275=CARTESIAN_POINT('Origin',(180.041252647846,81.7397376070391,299.047792462302));
#18276=CARTESIAN_POINT('Origin',(180.041252647846,81.7397376070391,299.047792462302));
#18277=CARTESIAN_POINT('Origin',(231.506382410955,81.7397376070391,298.714756191828));
#18278=CARTESIAN_POINT('Origin',(231.506382410955,81.7397376070391,298.714756191828));
#18279=CARTESIAN_POINT('Origin',(180.041252647846,81.7397376070391,305.073593133701));
#18280=CARTESIAN_POINT('Origin',(180.041252647846,81.7397376070391,339.073593133701));
#18281=CARTESIAN_POINT('Origin',(229.860277510589,81.7397376070391,311.321274222398));
#18282=CARTESIAN_POINT('Origin',(225.847649708814,81.7397376070391,342.051554365401));
#18283=CARTESIAN_POINT('Origin',(203.041252647846,81.7397376070391,339.073593133701));
#18284=CARTESIAN_POINT('Origin',(-292.274534377656,98.8263331110498,211.573593133701));
#18285=CARTESIAN_POINT('Ctrl Pts',(16.0838694668338,201.301935597134,215.573593133701));
#18286=CARTESIAN_POINT('Ctrl Pts',(15.9358379539975,201.392597584931,215.573593133701));
#18287=CARTESIAN_POINT('Ctrl Pts',(15.7937040698879,201.491453806169,215.566973449043));
#18288=CARTESIAN_POINT('Ctrl Pts',(15.4044650646298,201.796472278373,215.524024592965));
#18289=CARTESIAN_POINT('Ctrl Pts',(15.1550912170556,202.039779480087,215.462189646269));
#18290=CARTESIAN_POINT('Ctrl Pts',(14.7363053891028,202.553699758439,215.248657229881));
#18291=CARTESIAN_POINT('Ctrl Pts',(14.5662939349351,202.823424001646,215.095998687681));
#18292=CARTESIAN_POINT('Ctrl Pts',(14.3222646393754,203.293147538743,214.753756991984));
#18293=CARTESIAN_POINT('Ctrl Pts',(14.2316333870611,203.51606205111,214.554691098869));
#18294=CARTESIAN_POINT('Ctrl Pts',(14.1637727200979,203.720260967154,214.328111184109));
#18295=CARTESIAN_POINT('Origin',(-292.274534377656,98.8263331110498,294.573593133701));
#18296=CARTESIAN_POINT('Ctrl Pts',(14.1637727200979,203.720260967154,291.819075083293));
#18297=CARTESIAN_POINT('Ctrl Pts',(14.2316333870611,203.51606205111,291.592495168533));
#18298=CARTESIAN_POINT('Ctrl Pts',(14.3222646393754,203.293147538743,291.393429275417));
#18299=CARTESIAN_POINT('Ctrl Pts',(14.5662939349351,202.823424001646,291.05118757972));
#18300=CARTESIAN_POINT('Ctrl Pts',(14.7363053891028,202.553699758439,290.898529037521));
#18301=CARTESIAN_POINT('Ctrl Pts',(15.1550912170556,202.039779480087,290.684996621132));
#18302=CARTESIAN_POINT('Ctrl Pts',(15.4044650646298,201.796472278373,290.623161674437));
#18303=CARTESIAN_POINT('Ctrl Pts',(15.7937040698879,201.491453806169,290.580212818359));
#18304=CARTESIAN_POINT('Ctrl Pts',(15.9358379539975,201.392597584931,290.573593133701));
#18305=CARTESIAN_POINT('Ctrl Pts',(16.0838694668338,201.301935597134,290.573593133701));
#18306=CARTESIAN_POINT('Ctrl Pts',(-257.691868353317,110.319062001313,290.573593133701));
#18307=CARTESIAN_POINT('Ctrl Pts',(-257.226722972947,110.794866944168,290.573593133701));
#18308=CARTESIAN_POINT('Ctrl Pts',(-256.875952954917,111.37569206742,290.610062934072));
#18309=CARTESIAN_POINT('Ctrl Pts',(-256.575993830868,112.221556348799,290.839959190792));
#18310=CARTESIAN_POINT('Ctrl Pts',(-256.503984375586,112.507585568265,290.942908485374));
#18311=CARTESIAN_POINT('Ctrl Pts',(-256.419927726647,113.054277491751,291.217469046592));
#18312=CARTESIAN_POINT('Ctrl Pts',(-256.406892655266,113.314450931809,291.389750558212));
#18313=CARTESIAN_POINT('Ctrl Pts',(-256.416576787744,113.953138581935,291.926969681713));
#18314=CARTESIAN_POINT('Ctrl Pts',(-256.482778257329,114.307185871813,292.394274351607));
#18315=CARTESIAN_POINT('Ctrl Pts',(-256.596967428487,114.771542993549,293.443240125));
#18316=CARTESIAN_POINT('Ctrl Pts',(-256.639326258033,114.883947522592,294.024578076468));
#18317=CARTESIAN_POINT('Ctrl Pts',(-256.639326258033,114.883947522592,294.573593133701));
#18318=CARTESIAN_POINT('Origin',(-276.958747352154,36.7397376070391,217.573593133701));
#18319=CARTESIAN_POINT('Ctrl Pts',(262.041252647846,35.7397376070391,215.841542326132));
#18320=CARTESIAN_POINT('Ctrl Pts',(262.041252647846,35.8848665867868,215.757752070607));
#18321=CARTESIAN_POINT('Ctrl Pts',(262.058271315733,36.0525570221457,215.687285114485));
#18322=CARTESIAN_POINT('Ctrl Pts',(262.141705134945,36.3891914211257,215.596855314572));
#18323=CARTESIAN_POINT('Ctrl Pts',(262.208584003366,36.5579076658357,215.576473827892));
#18324=CARTESIAN_POINT('Ctrl Pts',(262.295835118638,36.7163102167537,215.573696499521));
#18325=CARTESIAN_POINT('Ctrl Pts',(262.302427956789,36.728004896672,215.573593133701));
#18326=CARTESIAN_POINT('Ctrl Pts',(262.309201840278,36.7397376070391,215.573593133701));
#18327=CARTESIAN_POINT('Ctrl Pts',(81.7733034554153,36.7397376070391,215.573593133701));
#18328=CARTESIAN_POINT('Ctrl Pts',(81.7800773389041,36.728004896672,215.573593133701));
#18329=CARTESIAN_POINT('Ctrl Pts',(81.7866701770546,36.7163102167537,215.573696499521));
#18330=CARTESIAN_POINT('Ctrl Pts',(81.8739212923264,36.5579076658357,215.576473827892));
#18331=CARTESIAN_POINT('Ctrl Pts',(81.9408001607482,36.3891914211257,215.596855314572));
#18332=CARTESIAN_POINT('Ctrl Pts',(82.0242339799602,36.0525570221457,215.687285114485));
#18333=CARTESIAN_POINT('Ctrl Pts',(82.0412526478464,35.8848665867869,215.757752070607));
#18334=CARTESIAN_POINT('Ctrl Pts',(82.0412526478464,35.7397376070391,215.841542326132));
#18335=CARTESIAN_POINT('Origin',(82.0412526478464,36.7397376070391,288.573593133701));
#18336=CARTESIAN_POINT('Ctrl Pts',(82.0412526478464,35.7397376070391,290.30564394127));
#18337=CARTESIAN_POINT('Ctrl Pts',(82.0412526478464,35.8848665867869,290.389434196794));
#18338=CARTESIAN_POINT('Ctrl Pts',(82.0242339799602,36.0525570221457,290.459901152916));
#18339=CARTESIAN_POINT('Ctrl Pts',(81.9408001607482,36.3891914211257,290.55033095283));
#18340=CARTESIAN_POINT('Ctrl Pts',(81.8739212923264,36.5579076658357,290.57071243951));
#18341=CARTESIAN_POINT('Ctrl Pts',(81.7866701770546,36.7163102167537,290.57348976788));
#18342=CARTESIAN_POINT('Ctrl Pts',(81.7800773389041,36.728004896672,290.573593133701));
#18343=CARTESIAN_POINT('Ctrl Pts',(81.7733034554153,36.7397376070391,290.573593133701));
#18344=CARTESIAN_POINT('Ctrl Pts',(262.309201840278,36.7397376070391,290.573593133701));
#18345=CARTESIAN_POINT('Ctrl Pts',(262.302427956789,36.728004896672,290.573593133701));
#18346=CARTESIAN_POINT('Ctrl Pts',(262.295835118638,36.7163102167537,290.57348976788));
#18347=CARTESIAN_POINT('Ctrl Pts',(262.208584003366,36.5579076658357,290.57071243951));
#18348=CARTESIAN_POINT('Ctrl Pts',(262.141705134945,36.3891914211257,290.55033095283));
#18349=CARTESIAN_POINT('Ctrl Pts',(262.058271315733,36.0525570221457,290.459901152916));
#18350=CARTESIAN_POINT('Ctrl Pts',(262.041252647846,35.8848665867869,290.389434196794));
#18351=CARTESIAN_POINT('Ctrl Pts',(262.041252647846,35.7397376070391,290.30564394127));
#18352=CARTESIAN_POINT('Origin',(-293.958747352154,39.7397376070391,203.073593133701));
#18353=CARTESIAN_POINT('Origin',(-293.958747352154,39.7397376070391,203.073593133701));
#18354=CARTESIAN_POINT('Origin',(-291.486115520766,96.4539090962284,297.073593133701));
#18355=CARTESIAN_POINT('Origin',(-291.486115520766,96.4539090962284,209.073593133701));
#18356=CARTESIAN_POINT('Origin',(-293.959747352154,39.7397376070391,303.073593133701));
#18357=CARTESIAN_POINT('Origin',(-293.959747352154,39.7397376070391,303.073593133701));
#18358=CARTESIAN_POINT('Ctrl Pts',(33.5102687927929,200.251018647718,288.573578335645));
#18359=CARTESIAN_POINT('Ctrl Pts',(33.5107199010858,200.251129484782,290.575563586967));
#18360=CARTESIAN_POINT('Ctrl Pts',(32.9669590743211,202.177851622247,290.573593109838));
#18361=CARTESIAN_POINT('Ctrl Pts',(34.0920283034919,200.415203421348,288.573424517396));
#18362=CARTESIAN_POINT('Ctrl Pts',(34.0347498209467,200.399019089839,290.421586252515));
#18363=CARTESIAN_POINT('Ctrl Pts',(33.6443849144762,202.203125958631,290.573595060035));
#18364=CARTESIAN_POINT('Ctrl Pts',(34.6840502924345,200.538691146292,288.592342587767));
#18365=CARTESIAN_POINT('Ctrl Pts',(34.6313932427609,200.529729997912,290.326885010332));
#18366=CARTESIAN_POINT('Ctrl Pts',(34.328746338229,202.221780639051,290.573596347446));
#18367=CARTESIAN_POINT('Ctrl Pts',(35.5864205375463,200.661622866077,288.615706152486));
#18368=CARTESIAN_POINT('Ctrl Pts',(35.5496884468174,200.657467722248,290.241178426705));
#18369=CARTESIAN_POINT('Ctrl Pts',(35.3681885540774,202.239169784339,290.573597581329));
#18370=CARTESIAN_POINT('Ctrl Pts',(35.8896886164042,200.692165047495,288.622846769446));
#18371=CARTESIAN_POINT('Ctrl Pts',(35.8596462675485,200.689666471269,290.22149043692));
#18372=CARTESIAN_POINT('Ctrl Pts',(35.716916186513,202.243194275642,290.573597875706));
#18373=CARTESIAN_POINT('Ctrl Pts',(36.4932960055171,200.731705119721,288.632640790062));
#18374=CARTESIAN_POINT('Ctrl Pts',(36.4764185460958,200.731103852825,290.196200221347));
#18375=CARTESIAN_POINT('Ctrl Pts',(36.4104416468938,202.247575398223,290.573598260089));
#18376=CARTESIAN_POINT('Ctrl Pts',(36.794514742425,200.740872444726,288.635321175873));
#18377=CARTESIAN_POINT('Ctrl Pts',(36.7867685126652,200.740894737748,290.190242235453));
#18378=CARTESIAN_POINT('Ctrl Pts',(36.7562545492582,202.247957465234,290.573598351964));
#18379=CARTESIAN_POINT('Ctrl Pts',(37.6964382193845,200.737132673354,288.635298337225));
#18380=CARTESIAN_POINT('Ctrl Pts',(37.7120443346043,200.737055769037,290.190295279034));
#18381=CARTESIAN_POINT('Ctrl Pts',(37.7918313998826,202.243752845543,290.573598351148));
#18382=CARTESIAN_POINT('Ctrl Pts',(38.2954125861561,200.693134716753,288.623593248778));
#18383=CARTESIAN_POINT('Ctrl Pts',(38.3371819114897,200.688812702912,290.213470083842));
#18384=CARTESIAN_POINT('Ctrl Pts',(38.4797294520679,202.233829054631,290.573597994748));
#18385=CARTESIAN_POINT('Ctrl Pts',(39.4912382499762,200.521128467222,288.592642194352));
#18386=CARTESIAN_POINT('Ctrl Pts',(39.5436846822378,200.511806765647,290.325533254215));
#18387=CARTESIAN_POINT('Ctrl Pts',(39.8584875384269,202.199733195285,290.573596366356));
#18388=CARTESIAN_POINT('Ctrl Pts',(40.0910570919123,200.391481338985,288.573422072675));
#18389=CARTESIAN_POINT('Ctrl Pts',(40.1485301709568,200.374739220995,290.421119323041));
#18390=CARTESIAN_POINT('Ctrl Pts',(40.5529097792499,202.175269274473,290.57359506633));
#18391=CARTESIAN_POINT('Ctrl Pts',(40.6733598348467,200.222036935988,288.573578350593));
#18392=CARTESIAN_POINT('Ctrl Pts',(40.6729077590008,200.222151960831,290.57556998517));
#18393=CARTESIAN_POINT('Ctrl Pts',(41.2322427580752,202.144417149988,290.57359310976));
#18394=CARTESIAN_POINT('Ctrl Pts',(40.6733364731919,200.222043778143,217.573607931757));
#18395=CARTESIAN_POINT('Ctrl Pts',(40.672886276363,200.222158261008,215.571622680597));
#18396=CARTESIAN_POINT('Ctrl Pts',(41.2322163763533,202.144418355354,215.573593157564));
#18397=CARTESIAN_POINT('Ctrl Pts',(40.0929242452915,200.390929578713,217.573761750004));
#18398=CARTESIAN_POINT('Ctrl Pts',(40.1500699231558,200.374282397278,215.725600014994));
#18399=CARTESIAN_POINT('Ctrl Pts',(40.5550171724534,202.175172199407,215.573591207367));
#18400=CARTESIAN_POINT('Ctrl Pts',(39.5019206382725,200.51920268524,217.554843679621));
#18401=CARTESIAN_POINT('Ctrl Pts',(39.5545034696285,200.509815837693,215.820301257091));
#18402=CARTESIAN_POINT('Ctrl Pts',(39.8708290592947,202.199362712531,215.573589919956));
#18403=CARTESIAN_POINT('Ctrl Pts',(38.6005744329249,200.649430503753,217.531480114922));
#18404=CARTESIAN_POINT('Ctrl Pts',(38.6372717067624,200.644978335475,215.906007840698));
#18405=CARTESIAN_POINT('Ctrl Pts',(38.8315615356453,202.225160314443,215.573588686073));
#18406=CARTESIAN_POINT('Ctrl Pts',(38.2975633626732,200.682425106419,217.524339497957));
#18407=CARTESIAN_POINT('Ctrl Pts',(38.3275845150866,200.679683571143,215.925695830483));
#18408=CARTESIAN_POINT('Ctrl Pts',(38.4828778729045,202.232005859847,215.573588391695));
#18409=CARTESIAN_POINT('Ctrl Pts',(37.6942956028995,200.726847032593,217.514545477341));
#18410=CARTESIAN_POINT('Ctrl Pts',(37.7111676458084,200.726109247728,215.950986046056));
#18411=CARTESIAN_POINT('Ctrl Pts',(37.7894105505436,202.241997418763,215.573588007313));
#18412=CARTESIAN_POINT('Ctrl Pts',(37.3931608862198,200.738450899264,217.511865091529));
#18413=CARTESIAN_POINT('Ctrl Pts',(37.4009070428415,200.73841052502,215.956944031954));
#18414=CARTESIAN_POINT('Ctrl Pts',(37.4436120554966,202.245177079077,215.573587915438));
#18415=CARTESIAN_POINT('Ctrl Pts',(36.4912366693717,200.742007757534,217.511887930177));
#18416=CARTESIAN_POINT('Ctrl Pts',(36.4756304426942,200.742057108271,215.95689098836));
#18417=CARTESIAN_POINT('Ctrl Pts',(36.4080350780731,202.249350352081,215.573587916253));
#18418=CARTESIAN_POINT('Ctrl Pts',(35.89192596265,200.702856907713,217.523593018625));
#18419=CARTESIAN_POINT('Ctrl Pts',(35.850123039343,200.698872946658,215.933716183589));
#18420=CARTESIAN_POINT('Ctrl Pts',(35.7200792538628,202.244991940212,215.573588272656));
#18421=CARTESIAN_POINT('Ctrl Pts',(34.6947479110263,200.540530445424,217.554544073045));
#18422=CARTESIAN_POINT('Ctrl Pts',(34.6422277830206,200.531633337413,215.821653013178));
#18423=CARTESIAN_POINT('Ctrl Pts',(34.3410904528754,202.22205126753,215.573589901044));
#18424=CARTESIAN_POINT('Ctrl Pts',(34.0938998602774,200.41574005857,217.573764194676));
#18425=CARTESIAN_POINT('Ctrl Pts',(34.0362932192499,200.399463442246,215.726066944493));
#18426=CARTESIAN_POINT('Ctrl Pts',(33.6464930249784,202.203205981858,215.573591201072));
#18427=CARTESIAN_POINT('Ctrl Pts',(33.5102453777233,200.251011995113,217.573607916811));
#18428=CARTESIAN_POINT('Ctrl Pts',(33.5106983692828,200.251123358914,215.571616282394));
#18429=CARTESIAN_POINT('Ctrl Pts',(32.9669326850786,202.177850630394,215.573593157641));
#18430=CARTESIAN_POINT('Origin',(179.041252647846,82.7397376070391,167.073593133701));
#18431=CARTESIAN_POINT('Origin',(226.839232189725,82.7397376070391,163.966155326709));
#18432=CARTESIAN_POINT('Origin',(179.041252647846,82.7397376070391,339.073593133701));
#18433=CARTESIAN_POINT('Origin',(179.041252647846,82.7397376070391,339.073593133701));
#18434=CARTESIAN_POINT('Origin',(203.041252647846,82.7397376070391,339.073593133701));
#18435=CARTESIAN_POINT('Origin',(226.839232189725,82.7397376070391,342.181030940692));
#18436=CARTESIAN_POINT('Origin',(233.091757762377,82.7397376070391,294.296733681953));
#18437=CARTESIAN_POINT('Origin',(80.0412526478464,35.7397376070391,295.073593133701));
#18438=CARTESIAN_POINT('Ctrl Pts',(82.0412526478464,35.7397376070391,294.996209423033));
#18439=CARTESIAN_POINT('Ctrl Pts',(82.0412526478464,35.9880846920539,295.034877011727));
#18440=CARTESIAN_POINT('Ctrl Pts',(81.9920100122073,36.2549156690397,295.0601656977));
#18441=CARTESIAN_POINT('Ctrl Pts',(81.8568715998261,36.5831910390556,295.072227252638));
#18442=CARTESIAN_POINT('Ctrl Pts',(81.8175214272437,36.6631498332247,295.073593133701));
#18443=CARTESIAN_POINT('Ctrl Pts',(81.7733034554153,36.7397376070391,295.073593133701));
#18444=CARTESIAN_POINT('Origin',(80.0412526478464,35.7397376070391,211.073593133701));
#18445=CARTESIAN_POINT('Ctrl Pts',(81.7733034554153,36.7397376070391,211.073593133701));
#18446=CARTESIAN_POINT('Ctrl Pts',(81.8175214272437,36.6631498332247,211.073593133701));
#18447=CARTESIAN_POINT('Ctrl Pts',(81.8568715998261,36.5831910390556,211.074959014763));
#18448=CARTESIAN_POINT('Ctrl Pts',(81.9920100122073,36.2549156690397,211.087020569701));
#18449=CARTESIAN_POINT('Ctrl Pts',(82.0412526478464,35.9880846920539,211.112309255674));
#18450=CARTESIAN_POINT('Ctrl Pts',(82.0412526478464,35.7397376070391,211.150976844368));
#18451=CARTESIAN_POINT('Origin',(264.041252647846,35.7397376070391,253.073593133701));
#18452=CARTESIAN_POINT('Ctrl Pts',(262.041252647846,35.7397376070391,211.150976844368));
#18453=CARTESIAN_POINT('Ctrl Pts',(262.041252647846,35.9880846920539,211.112309255674));
#18454=CARTESIAN_POINT('Ctrl Pts',(262.090495283485,36.2549156690397,211.087020569701));
#18455=CARTESIAN_POINT('Ctrl Pts',(262.225633695867,36.5831910390556,211.074959014763));
#18456=CARTESIAN_POINT('Ctrl Pts',(262.264983868449,36.6631498332246,211.073593133701));
#18457=CARTESIAN_POINT('Ctrl Pts',(262.309201840278,36.7397376070391,211.073593133701));
#18458=CARTESIAN_POINT('Origin',(264.041252647846,35.7397376070391,253.073593133701));
#18459=CARTESIAN_POINT('Ctrl Pts',(262.309201840278,36.7397376070391,295.073593133701));
#18460=CARTESIAN_POINT('Ctrl Pts',(262.264983868449,36.6631498332247,295.073593133701));
#18461=CARTESIAN_POINT('Ctrl Pts',(262.225633695867,36.5831910390556,295.072227252638));
#18462=CARTESIAN_POINT('Ctrl Pts',(262.090495283485,36.2549156690397,295.0601656977));
#18463=CARTESIAN_POINT('Ctrl Pts',(262.041252647846,35.9880846920539,295.034877011727));
#18464=CARTESIAN_POINT('Ctrl Pts',(262.041252647846,35.7397376070391,294.996209423033));
#18465=CARTESIAN_POINT('Origin',(-260.909689484712,113.464793580191,253.073593133701));
#18466=CARTESIAN_POINT('Origin',(18.4341359467765,205.139414909555,211.073593133701));
#18467=CARTESIAN_POINT('Origin',(18.4341359467765,205.139414909555,295.073593133701));
#18468=CARTESIAN_POINT('Origin',(-276.958747352154,36.7397376070391,288.573593133701));
#18469=CARTESIAN_POINT('Origin',(82.0412526478464,36.7397376070391,217.573593133701));
#27751=UNCERTAINTY_MEASURE_WITH_UNIT(LENGTH_MEASURE(0.01),#27808,
'DISTANCE_ACCURACY_VALUE',
'Maximum model space distance between geometric entities at asserted c
onnectivities');
#27778=UNCERTAINTY_MEASURE_WITH_UNIT(LENGTH_MEASURE(0.01),#27808,
'DISTANCE_ACCURACY_VALUE',
'Maximum model space distance between geometric entities at asserted c
onnectivities');
#27780=(
GEOMETRIC_REPRESENTATION_CONTEXT(3)
GLOBAL_UNCERTAINTY_ASSIGNED_CONTEXT((#27751))
GLOBAL_UNIT_ASSIGNED_CONTEXT((#27808,#27810,#27811))
REPRESENTATION_CONTEXT('','3D')
);
#27807=(
GEOMETRIC_REPRESENTATION_CONTEXT(3)
GLOBAL_UNCERTAINTY_ASSIGNED_CONTEXT((#27778))
GLOBAL_UNIT_ASSIGNED_CONTEXT((#27808,#27810,#27811))
REPRESENTATION_CONTEXT('','3D')
);
#27808=(
LENGTH_UNIT()
NAMED_UNIT(*)
SI_UNIT(.MILLI.,.METRE.)
);
#27810=(
NAMED_UNIT(*)
PLANE_ANGLE_UNIT()
SI_UNIT($,.RADIAN.)
);
#27811=(
NAMED_UNIT(*)
SI_UNIT($,.STERADIAN.)
SOLID_ANGLE_UNIT()
);
#27813=SHAPE_DEFINITION_REPRESENTATION(#27841,#27900);
#27841=PRODUCT_DEFINITION_SHAPE('',$,#27929);
#27900=SHAPE_REPRESENTATION('',(#12299),#27780);
#27927=PRODUCT_DEFINITION_CONTEXT('part definition',#28013,'design');
#27929=PRODUCT_DEFINITION('Main Frame','Main Frame',#27957,#27927);
#27957=PRODUCT_DEFINITION_FORMATION('',$,#28016);
#28013=APPLICATION_CONTEXT('Managed model based 3d engineering');
#28014=PRODUCT_CONTEXT('part definition',#28013,'mechanical');
#28016=PRODUCT('Main Frame','Main Frame',$,(#28014));
#28050=COLOUR_RGB('Dark Blue',0.08,0.2,0.34);
#28051=FILL_AREA_STYLE_COLOUR('',#28050);
#28052=FILL_AREA_STYLE('',(#28051));
#28053=SURFACE_STYLE_FILL_AREA(#28052);
#28054=SURFACE_SIDE_STYLE('',(#28053));
#28055=SURFACE_STYLE_USAGE(.BOTH.,#28054);
#28056=PRESENTATION_STYLE_ASSIGNMENT((#28055));
ENDSEC;
END-ISO-10303-21;
